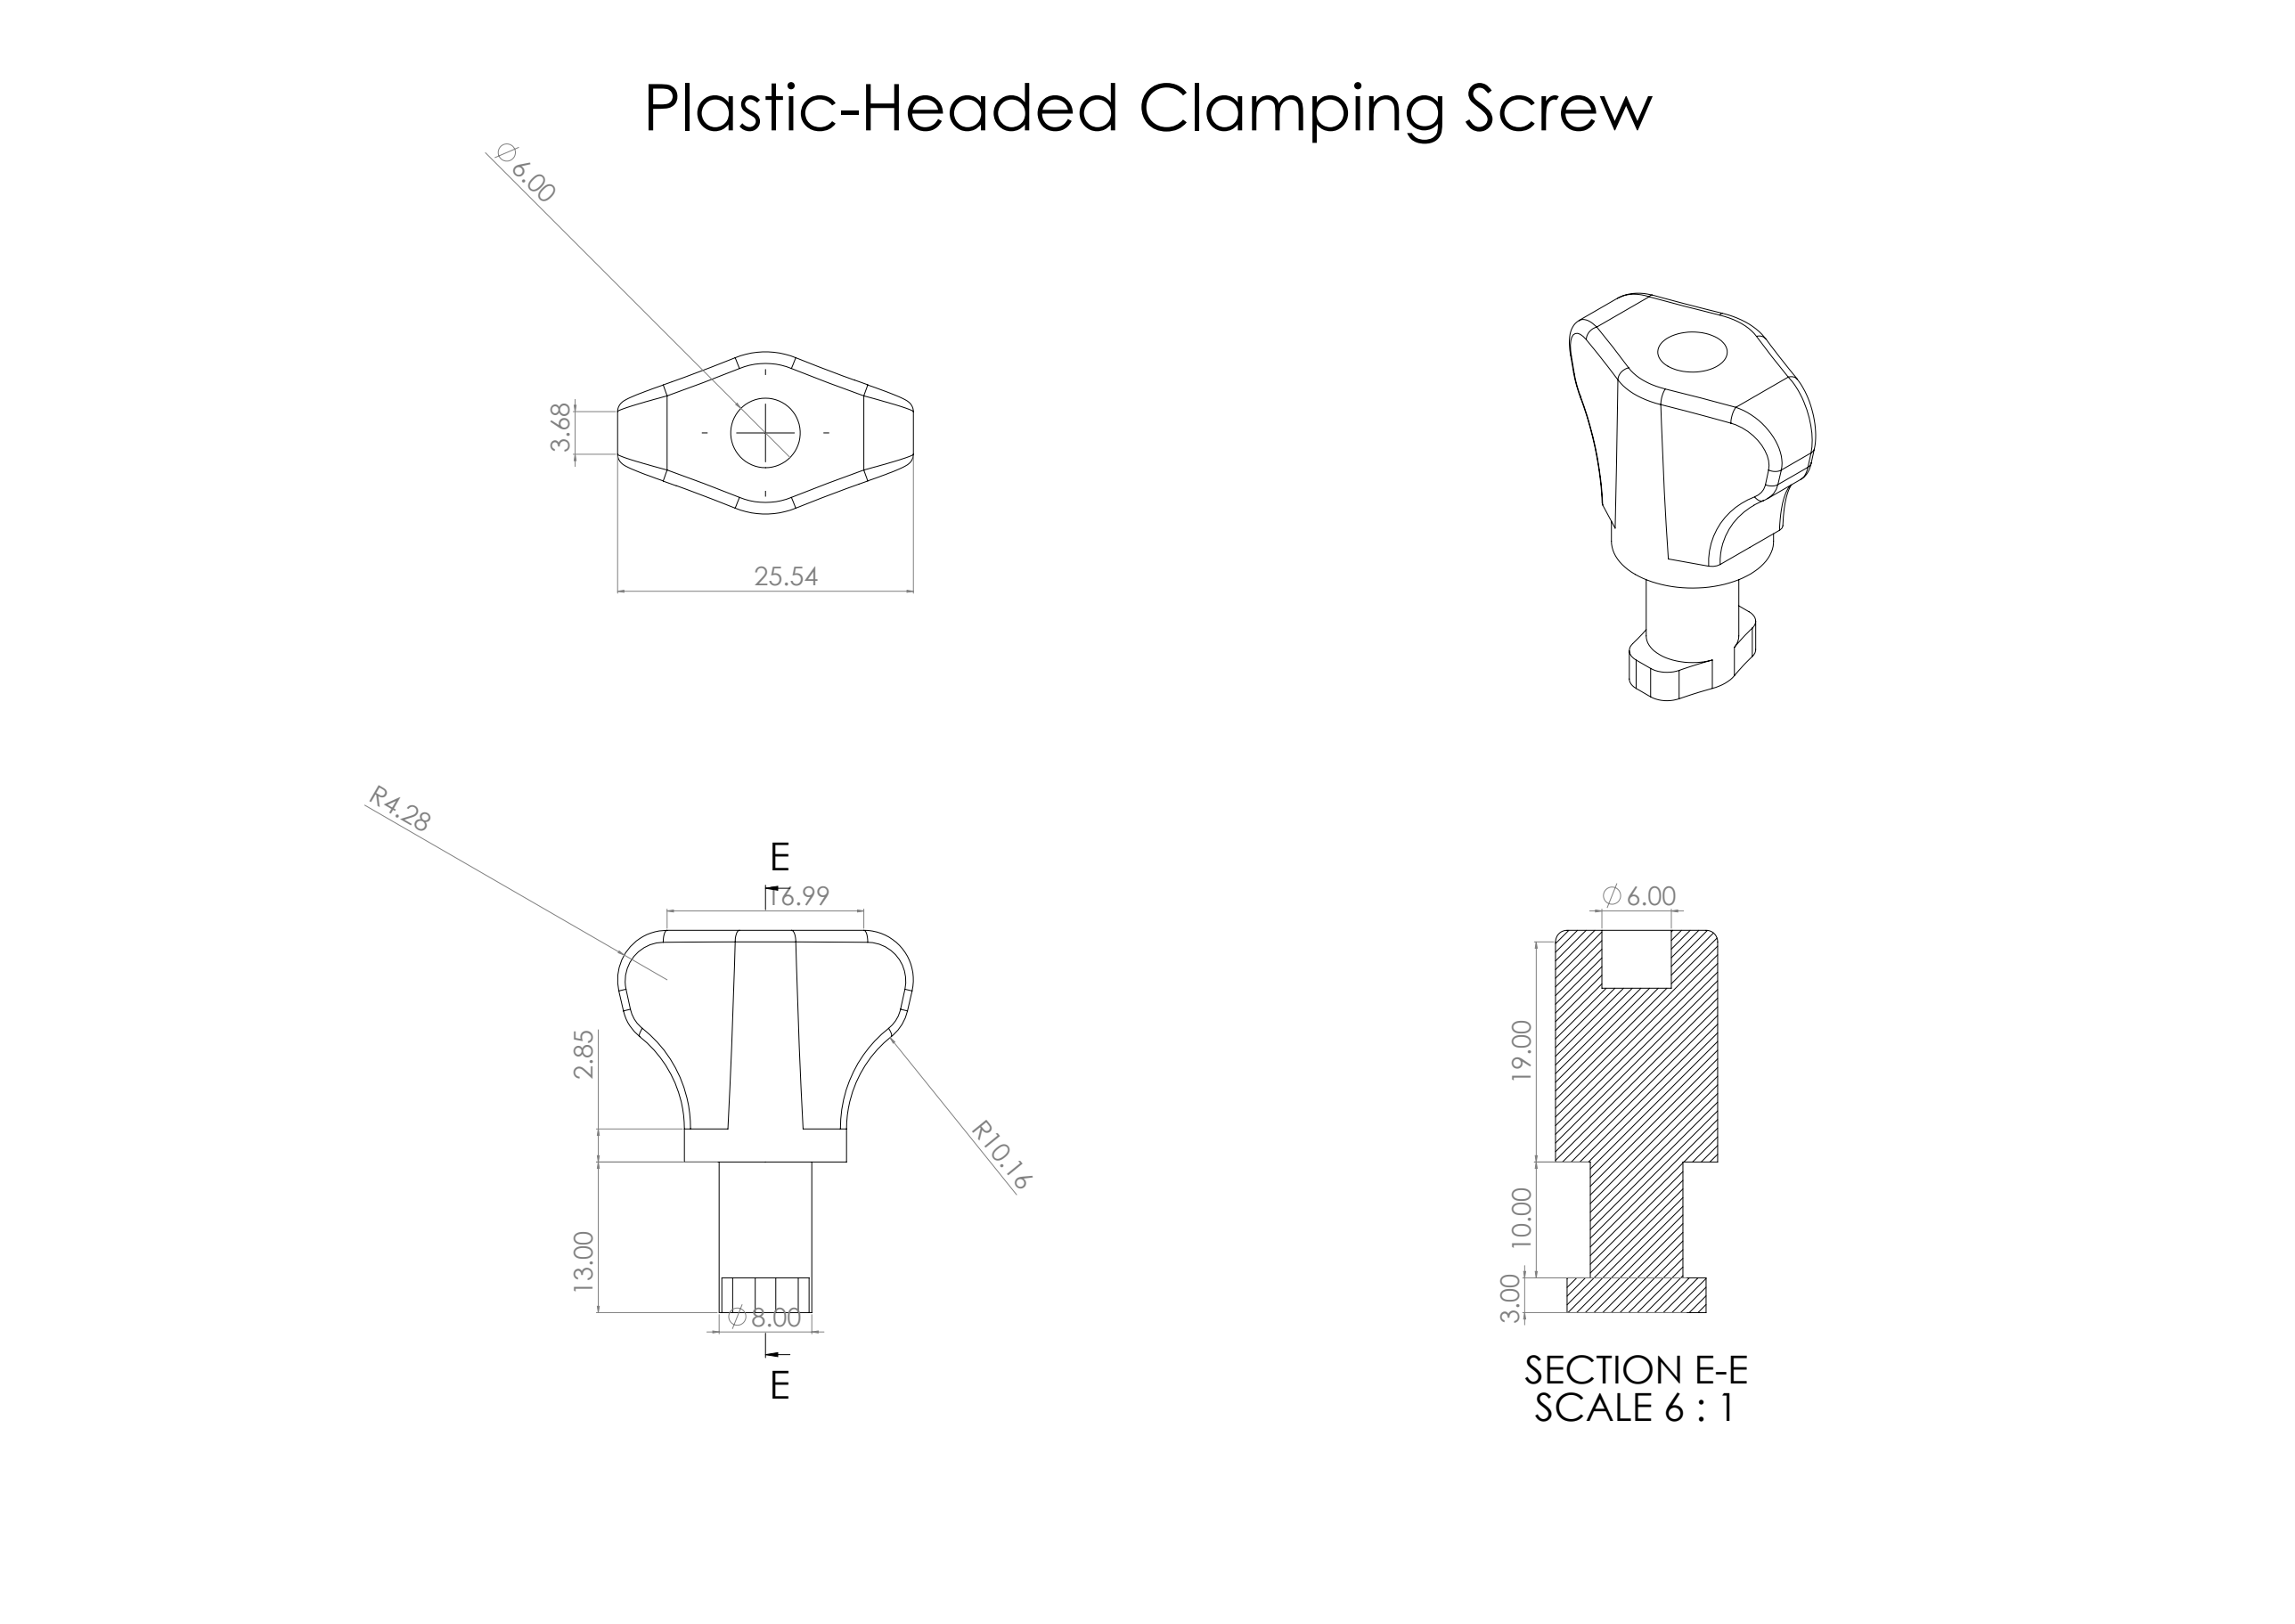
ISO-10303-21;
HEADER;
FILE_DESCRIPTION (('STEP AP214'),
    '1' );
FILE_NAME ('Plastic-Headed Clamping Screw.step',
    '2026-10-24T21:31:31',
    ( '' ),
    ( '' ),
    'SwSTEP 2.0',
    'SolidWorks 2025',
    '' );
FILE_SCHEMA (( 'AUTOMOTIVE_DESIGN' ));
ENDSEC;

DATA;
#4=EDGE_CURVE ( 'NONE', #12159, #10942, #11483, .T. ) ;
#5=EDGE_LOOP ( 'NONE', ( #6099, #8745, #4266, #9000 ) ) ;
#9=CARTESIAN_POINT ( 'NONE',  ( 27.62489819272141389, -52.24929059928630437, 4.899481419381555014 ) ) ;
#10=CARTESIAN_POINT ( 'NONE',  ( 23.72005712271873890, -60.79495753911086098, 6.390225278796987318 ) ) ;
#18=ADVANCED_FACE ( 'NONE', ( #1362 ), #5786, .T. ) ;
#24=ORIENTED_EDGE ( 'NONE', *, *, #9295, .T. ) ;
#52=CARTESIAN_POINT ( 'NONE',  ( 8.091875466796944139, -56.52532528994245808, 1.842181053809107238 ) ) ;
#55=EDGE_CURVE ( 'NONE', #10251, #7651, #14932, .T. ) ;
#67=CARTESIAN_POINT ( 'NONE',  ( 8.466388902489018875, -58.63671300496866223, -1.826958383930360919 ) ) ;
#70=CIRCLE ( 'NONE', #4772, 3.000000000000000888 ) ;
#78=CARTESIAN_POINT ( 'NONE',  ( 10.10272221478045296, -60.61171897230391892, -3.004288329735573804 ) ) ;
#82=B_SPLINE_CURVE_WITH_KNOTS ( 'NONE', 3,
 ( #2803, #3028, #1934, #12180, #8712, #1641, #3094, #13404, #11248, #10961, #410, #7643, #1857, #1791, #7796, #12259, #700, #6406 ),
 .UNSPECIFIED., .F., .F.,
 ( 4, 2, 2, 2, 2, 2, 2, 2, 4 ),
 ( 0.000000000000000000, 0.0007600084067931386217, 0.001520016813586277243, 0.002280025220379415865, 0.003040033627172554487, 0.003800042033965693108, 0.004560050440758831730, 0.005320058847551970352, 0.006080067254345108974 ),
 .UNSPECIFIED. ) ;
#88=FACE_OUTER_BOUND ( 'NONE', #4233, .T. ) ;
#89=ORIENTED_EDGE ( 'NONE', *, *, #5308, .T. ) ;
#91=CARTESIAN_POINT ( 'NONE',  ( 32.77533487224304309, -57.91121052158847249, 2.751677492798574320 ) ) ;
#95=VECTOR ( 'NONE', #9996, 1000.000000000000000 ) ;
#96=DIRECTION ( 'NONE',  ( 0.9421718071228325497, 6.170304995646513309E-16, -0.3351302520855077849 ) ) ;
#102=ORIENTED_EDGE ( 'NONE', *, *, #10358, .T. ) ;
#104=CARTESIAN_POINT ( 'NONE',  ( 9.074528850127588697, -58.48798588983633095, 2.754379989674547780 ) ) ;
#112=EDGE_CURVE ( 'NONE', #12771, #10151, #4658, .T. ) ;
#113=CARTESIAN_POINT ( 'NONE',  ( 33.37135420079148673, -55.04126158147273884, -2.748788379873860599 ) ) ;
#125=CARTESIAN_POINT ( 'NONE',  ( 13.86797143582180780, -68.67521603617343828, 4.260811380360699729 ) ) ;
#126=DIRECTION ( 'NONE',  ( 0.000000000000000000, 0.000000000000000000, 1.000000000000000000 ) ) ;
#129=CARTESIAN_POINT ( 'NONE',  ( 30.58625090343030806, -52.41844408481608752, 2.861639392408844351 ) ) ;
#131=CARTESIAN_POINT ( 'NONE',  ( 20.86173033120691045, -53.24929059928630437, 0.000000000000000000 ) ) ;
#139=CARTESIAN_POINT ( 'NONE',  ( 9.123957934261133218, -53.72645478541605257, 3.103403305059656336 ) ) ;
#143=VERTEX_POINT ( 'NONE', #9046 ) ;
#146=DIRECTION ( 'NONE',  ( -0.9744556954135545901, 0.2245798247307304318, 0.000000000000000000 ) ) ;
#173=CARTESIAN_POINT ( 'NONE',  ( 29.24198010098110245, -64.22824823034754615, 3.135769320951033112 ) ) ;
#174=EDGE_CURVE ( 'NONE', #2378, #7934, #12219, .T. ) ;
#176=CARTESIAN_POINT ( 'NONE',  ( 13.73779544508787431, -66.12426320349668174, 4.110478850042866839 ) ) ;
#180=CARTESIAN_POINT ( 'NONE',  ( 33.55553634841081845, -55.70626543767114214, 1.910065177037574946 ) ) ;
#188=CARTESIAN_POINT ( 'NONE',  ( 18.24487436548682240, -53.24929059928630437, 6.492462156583986399 ) ) ;
#201=CARTESIAN_POINT ( 'NONE',  ( 32.69801279946867112, -53.84541978742783641, 3.062363702218897643 ) ) ;
#226=CYLINDRICAL_SURFACE ( 'NONE', #7156, 10.15857703477299978 ) ;
#228=CARTESIAN_POINT ( 'NONE',  ( 12.36791015745245836, -52.24929059928630437, 3.199931146564424012 ) ) ;
#234=ORIENTED_EDGE ( 'NONE', *, *, #174, .T. ) ;
#239=CARTESIAN_POINT ( 'NONE',  ( 24.10826840236109803, -69.39711819508849544, -6.201611931792124111 ) ) ;
#256=CARTESIAN_POINT ( 'NONE',  ( 9.949736305181877682, -63.13800426656748499, 2.713090553606876121 ) ) ;
#258=CARTESIAN_POINT ( 'NONE',  ( 27.33382790127958728, -69.39711819508849544, 4.502057496415716287 ) ) ;
#259=DIRECTION ( 'NONE',  ( 0.000000000000000000, 0.000000000000000000, 1.000000000000000000 ) ) ;
#261=CARTESIAN_POINT ( 'NONE',  ( 31.94014848486111191, -53.10528739703779877, -3.364210193422788375 ) ) ;
#264=EDGE_CURVE ( 'NONE', #12856, #5130, #362, .T. ) ;
#266=DIRECTION ( 'NONE',  ( -0.000000000000000000, -0.000000000000000000, -1.000000000000000000 ) ) ;
#276=CARTESIAN_POINT ( 'NONE',  ( 31.87918814257875155, -54.14181112192009238, 3.331498666157771016 ) ) ;
#289=CARTESIAN_POINT ( 'NONE',  ( 9.168176149879958103, -53.68423722363644401, 2.283982087543965367 ) ) ;
#300=ORIENTED_EDGE ( 'NONE', *, *, #12912, .T. ) ;
#301=CARTESIAN_POINT ( 'NONE',  ( 13.63336148250377100, -65.27414832489905905, 4.302972696997120039 ) ) ;
#302=VERTEX_POINT ( 'NONE', #4387 ) ;
#304=VERTEX_POINT ( 'NONE', #7858 ) ;
#308=AXIS2_PLACEMENT_3D ( 'NONE', #9751, #6496, #11257 ) ;
#309=ADVANCED_FACE ( 'NONE', ( #12548, #6765 ), #13774, .T. ) ;
#312=CARTESIAN_POINT ( 'NONE',  ( 29.48535251946101710, -62.76259148841303670, -3.786770376139251937 ) ) ;
#314=ORIENTED_EDGE ( 'NONE', *, *, #11289, .T. ) ;
#316=CARTESIAN_POINT ( 'NONE',  ( 32.90197589884652274, -57.33450387999030795, 2.749014434309885235 ) ) ;
#325=ORIENTED_EDGE ( 'NONE', *, *, #6325, .F. ) ;
#330=CARTESIAN_POINT ( 'NONE',  ( 13.85027004230004444, -68.05254135517340330, 4.069129116404105240 ) ) ;
#331=CARTESIAN_POINT ( 'NONE',  ( 32.35433946108159375, -60.80954383512729322, 1.970170733381438222 ) ) ;
#332=VECTOR ( 'NONE', #3067, 1000.000000000000000 ) ;
#333=CARTESIAN_POINT ( 'NONE',  ( 12.03298173962126683, -53.28399145779480506, 4.141535524925028078 ) ) ;
#338=CARTESIAN_POINT ( 'NONE',  ( 32.37230692610057758, -54.69057383521065674, -3.126673503084364203 ) ) ;
#343=DIRECTION ( 'NONE',  ( 0.9744556954135530358, -0.2245798247307378148, 0.000000000000000000 ) ) ;
#362=B_SPLINE_CURVE_WITH_KNOTS ( 'NONE', 3,
 ( #5026, #12249, #5902, #7328, #3856, #12016, #331, #8559, #13257, #9804 ),
 .UNSPECIFIED., .F., .F.,
 ( 4, 2, 2, 2, 4 ),
 ( 0.000000000000000000, 0.0006693228878568694860, 0.001338645775713738972, 0.002007968663570608350, 0.002677291551427477944 ),
 .UNSPECIFIED. ) ;
#374=CARTESIAN_POINT ( 'NONE',  ( 31.12893072306533071, -61.89517205450268733, 2.369674354374375458 ) ) ;
#378=EDGE_LOOP ( 'NONE', ( #12434, #11503, #11290, #1533 ) ) ;
#383=CARTESIAN_POINT ( 'NONE',  ( 19.97461805067967688, 0.000000000000000000, -4.000000000000000888 ) ) ;
#399=CARTESIAN_POINT ( 'NONE',  ( 31.74193665722908264, -52.96285630328479499, 2.532360049841041683 ) ) ;
#407=DIRECTION ( 'NONE',  ( 0.000000000000000000, 0.000000000000000000, 1.000000000000000000 ) ) ;
#410=CARTESIAN_POINT ( 'NONE',  ( 9.212626894557791601, -54.90380519981211194, 3.064473585392920363 ) ) ;
#414=CARTESIAN_POINT ( 'NONE',  ( 27.86173033120691045, -69.39711819508849544, -3.619682905202609380 ) ) ;
#418=ORIENTED_EDGE ( 'NONE', *, *, #1578, .T. ) ;
#420=CARTESIAN_POINT ( 'NONE',  ( 28.47348575918184110, -58.78531205411836424, -4.199849437517832129 ) ) ;
#424=DIRECTION ( 'NONE',  ( 0.000000000000000000, 0.000000000000000000, -1.000000000000000000 ) ) ;
#425=DIRECTION ( 'NONE',  ( 0.000000000000000000, -1.000000000000000000, 0.000000000000000000 ) ) ;
#427=ORIENTED_EDGE ( 'NONE', *, *, #10079, .F. ) ;
#430=ADVANCED_FACE ( 'NONE', ( #12701 ), #5856, .T. ) ;
#432=CYLINDRICAL_SURFACE ( 'NONE', #9177, 3.951771890309582869 ) ;
#439=LINE ( 'NONE', #4985, #3268 ) ;
#447=CARTESIAN_POINT ( 'NONE',  ( 28.71810018070638648, -65.29678988936899486, 3.348867343503173721 ) ) ;
#448=ADVANCED_FACE ( 'NONE', ( #7159 ), #15184, .T. ) ;
#462=ORIENTED_EDGE ( 'NONE', *, *, #9510, .T. ) ;
#463=EDGE_LOOP ( 'NONE', ( #8239, #3179, #633, #6797, #6640 ) ) ;
#468=( BOUNDED_SURFACE ( )  B_SPLINE_SURFACE ( 3, 2, ( 
 ( #9739, #10958, #7416 ),
 ( #11029, #14423, #4081 ),
 ( #12112, #6268, #3867 ),
 ( #14564, #12255, #11095 ) ),
 .UNSPECIFIED., .F., .F., .F. ) 
 B_SPLINE_SURFACE_WITH_KNOTS ( ( 4, 4 ),
 ( 3, 3 ),
 ( 0.000000000000000000, 0.001771943201165730557 ),
 ( 0.000000000000000000, 1.000000000000000000 ),
 .UNSPECIFIED. ) 
 GEOMETRIC_REPRESENTATION_ITEM ( )  RATIONAL_B_SPLINE_SURFACE ( (
 ( 1.000000000000000000, 0.8308543624379411963, 1.000000000000000000),
 ( 1.000000000000000000, 0.8288551047899443969, 1.000000000000000000),
 ( 1.000000000000000000, 0.8269348987755755775, 1.000000000000000000),
 ( 1.000000000000000000, 0.8250833044923659987, 1.000000000000000000) ) ) 
 REPRESENTATION_ITEM ( '' )  SURFACE ( )  );
#470=CARTESIAN_POINT ( 'NONE',  ( 10.05209847106513621, -63.64501252278640919, 2.710939438195351325 ) ) ;
#474=CARTESIAN_POINT ( 'NONE',  ( 13.86142555056148851, -69.48056866272027321, -4.214447830835809761 ) ) ;
#484=DIRECTION ( 'NONE',  ( 0.3351302520855081735, 0.000000000000000000, -0.9421718071228324387 ) ) ;
#500=CARTESIAN_POINT ( 'NONE',  ( 29.27360327072251067, -58.32476007869853873, 2.500000000000000000 ) ) ;
#502=CARTESIAN_POINT ( 'NONE',  ( 20.86173033120691045, -72.24929059928631148, 3.999999999999999112 ) ) ;
#508=AXIS2_PLACEMENT_3D ( 'NONE', #2758, #1819, #6294 ) ;
#512=CARTESIAN_POINT ( 'NONE',  ( 27.33509234239454244, -69.49659648540917090, 4.497058153269692937 ) ) ;
#544=CARTESIAN_POINT ( 'NONE',  ( 10.45251858056743011, -61.76394201830515129, -3.065891788180099553 ) ) ;
#552=DIRECTION ( 'NONE',  ( -0.2245798247307348172, -0.9744556954135535909, 0.000000000000000000 ) ) ;
#554=( NAMED_UNIT ( * ) PLANE_ANGLE_UNIT ( ) SI_UNIT ( $, .RADIAN. ) );
#564=CARTESIAN_POINT ( 'NONE',  ( 20.86173033120691045, -57.24929059928630437, 0.000000000000000000 ) ) ;
#567=CARTESIAN_POINT ( 'NONE',  ( 23.50212160826626118, -54.09900330347249309, -6.482993899729486920 ) ) ;
#572=DIRECTION ( 'NONE',  ( 0.000000000000000000, 0.000000000000000000, -1.000000000000000000 ) ) ;
#574=ORIENTED_EDGE ( 'NONE', *, *, #3154, .F. ) ;
#579=CARTESIAN_POINT ( 'NONE',  ( 11.75462132594869047, -63.18892729117109042, 3.546101824479054976 ) ) ;
#580=EDGE_CURVE ( 'NONE', #13749, #4765, #2911, .T. ) ;
#581=CARTESIAN_POINT ( 'NONE',  ( 11.41483174849314786, -52.33251913750716255, 3.960984348906031460 ) ) ;
#585=FACE_OUTER_BOUND ( 'NONE', #3678, .T. ) ;
#598=FACE_OUTER_BOUND ( 'NONE', #463, .T. ) ;
#599=CYLINDRICAL_SURFACE ( 'NONE', #8676, 10.15857703477299623 ) ;
#611=CARTESIAN_POINT ( 'NONE',  ( 8.749277640414614865, -56.32592369292856915, -2.799485268159552120 ) ) ;
#615=CARTESIAN_POINT ( 'NONE',  ( 14.40311142432127056, -68.64054039872911517, -4.542265185092021262 ) ) ;
#617=CARTESIAN_POINT ( 'NONE',  ( 33.62912904389242641, -56.86646964060239640, 2.513983171436027231 ) ) ;
#621=FACE_OUTER_BOUND ( 'NONE', #8917, .T. ) ;
#622=EDGE_CURVE ( 'NONE', #15091, #1508, #10780, .T. ) ;
#624=CARTESIAN_POINT ( 'NONE',  ( 9.200644618036296407, -59.06479067038043240, -2.757123406423053424 ) ) ;
#625=VERTEX_POINT ( 'NONE', #1612 ) ;
#627=CARTESIAN_POINT ( 'NONE',  ( 27.86173033120691045, -69.39711819508848123, -3.801276035476822468 ) ) ;
#632=CARTESIAN_POINT ( 'NONE',  ( 28.15780090692999593, -63.36830850591302067, -4.156137255743351133 ) ) ;
#633=ORIENTED_EDGE ( 'NONE', *, *, #14074, .F. ) ;
#640=CIRCLE ( 'NONE', #11212, 0.9999999999999996669 ) ;
#643=CARTESIAN_POINT ( 'NONE',  ( 31.33007899711186894, -52.72918400488543256, -2.651310087704546348 ) ) ;
#651=AXIS2_PLACEMENT_3D ( 'NONE', #8278, #11802, #11951 ) ;
#652=DIRECTION ( 'NONE',  ( 0.000000000000000000, 0.000000000000000000, -1.000000000000000000 ) ) ;
#656=EDGE_LOOP ( 'NONE', ( #5765, #14402, #234, #3280, #10430, #12233, #7508, #462, #7848 ) ) ;
#658=B_SPLINE_CURVE_WITH_KNOTS ( 'NONE', 3,
 ( #10135, #10365, #13747, #3202 ),
 .UNSPECIFIED., .F., .F.,
 ( 4, 4 ),
 ( 0.000000000000000000, 0.001771361151111829372 ),
 .UNSPECIFIED. ) ;
#662=ORIENTED_EDGE ( 'NONE', *, *, #7032, .T. ) ;
#666=ORIENTED_EDGE ( 'NONE', *, *, #12524, .F. ) ;
#668=CARTESIAN_POINT ( 'NONE',  ( 11.71690433395004227, -52.27452423507673274, -4.068013018868786190 ) ) ;
#669=DIRECTION ( 'NONE',  ( -0.6198786537240911221, -0.7846976836063734861, 0.000000000000000000 ) ) ;
#672=ORIENTED_EDGE ( 'NONE', *, *, #12291, .F. ) ;
#680=CARTESIAN_POINT ( 'NONE',  ( 8.597635011448854669, -59.20619211347771227, -2.502190571104482952 ) ) ;
#684=EDGE_CURVE ( 'NONE', #12779, #2517, #9724, .T. ) ;
#688=CARTESIAN_POINT ( 'NONE',  ( 12.06814882729969440, -63.62021712492819603, -2.966460067268481549 ) ) ;
#694=ORIENTED_EDGE ( 'NONE', *, *, #1475, .T. ) ;
#700=CARTESIAN_POINT ( 'NONE',  ( 8.766252841628377368, -57.08298494442340143, 2.747852995220871009 ) ) ;
#701=CARTESIAN_POINT ( 'NONE',  ( 10.00023835250150483, -61.42570632716525125, 2.132522520905371977 ) ) ;
#704=AXIS2_PLACEMENT_3D ( 'NONE', #10886, #8709, #343 ) ;
#710=ORIENTED_EDGE ( 'NONE', *, *, #1180, .T. ) ;
#716=CARTESIAN_POINT ( 'NONE',  ( 14.22956937301584546, -69.39711819508849544, -4.416273062436609109 ) ) ;
#720=CARTESIAN_POINT ( 'NONE',  ( 8.649830367478799076, -59.43266865480772054, -1.834006918418332521 ) ) ;
#728=DIRECTION ( 'NONE',  ( 0.000000000000000000, 1.000000000000000000, 0.000000000000000000 ) ) ;
#736=ORIENTED_EDGE ( 'NONE', *, *, #1578, .F. ) ;
#743=DIRECTION ( 'NONE',  ( -0.000000000000000000, -0.000000000000000000, -1.000000000000000000 ) ) ;
#753=EDGE_CURVE ( 'NONE', #12307, #1292, #9416, .T. ) ;
#759=LINE ( 'NONE', #8997, #13503 ) ;
#764=CARTESIAN_POINT ( 'NONE',  ( 15.46081644285382772, -69.39711819508849544, 5.076148092048922145 ) ) ;
#768=CARTESIAN_POINT ( 'NONE',  ( 32.90197589884652274, -57.33450387999031506, 2.749014434309864363 ) ) ;
#773=CARTESIAN_POINT ( 'NONE',  ( 29.49975272800921289, -62.74348037527474276, -3.781439773221457301 ) ) ;
#783=CARTESIAN_POINT ( 'NONE',  ( 32.95707784766408110, -57.08357682498795072, 2.747855728348003179 ) ) ;
#790=CIRCLE ( 'NONE', #3744, 2.000000000000000000 ) ;
#792=CARTESIAN_POINT ( 'NONE',  ( 20.86173033120691045, -57.24929059928630437, 3.000000000000000888 ) ) ;
#797=CIRCLE ( 'NONE', #14087, 1.000000000000001332 ) ;
#798=CARTESIAN_POINT ( 'NONE',  ( 13.51972775594646947, -66.75404937493283342, 3.551013195535614120 ) ) ;
#801=CARTESIAN_POINT ( 'NONE',  ( 33.59633122631266389, -57.16466038563396523, -1.814534822646767909 ) ) ;
#808=CARTESIAN_POINT ( 'NONE',  ( 7.497055383622185154, -51.17811635675307969, -2.733205671937324777 ) ) ;
#811=ORIENTED_EDGE ( 'NONE', *, *, #7029, .T. ) ;
#814=ADVANCED_FACE ( 'NONE', ( #10570 ), #5184, .T. ) ;
#816=DIRECTION ( 'NONE',  ( 0.000000000000000000, 0.000000000000000000, -1.000000000000000000 ) ) ;
#822=CARTESIAN_POINT ( 'NONE',  ( 8.605785544313173219, -54.47948885957401188, -2.876625435111462625 ) ) ;
#829=EDGE_LOOP ( 'NONE', ( #10229, #6980, #7558, #1341 ) ) ;
#832=EDGE_LOOP ( 'NONE', ( #908, #9068, #8291, #12526 ) ) ;
#834=FACE_OUTER_BOUND ( 'NONE', #12615, .T. ) ;
#835=CARTESIAN_POINT ( 'NONE',  ( 10.21509949969620834, -53.84182990103197142, -3.477143273224481579 ) ) ;
#840=CARTESIAN_POINT ( 'NONE',  ( 32.90197589884652274, -57.33450387999030085, -2.749014434309871024 ) ) ;
#843=ADVANCED_FACE ( 'NONE', ( #8557 ), #10988, .F. ) ;
#849=CARTESIAN_POINT ( 'NONE',  ( 27.69711443911335991, -66.46764508687284945, -4.441229594909795964 ) ) ;
#853=B_SPLINE_CURVE_WITH_KNOTS ( 'NONE', 3,
 ( #870, #3338, #5576, #8037, #7337, #2342 ),
 .UNSPECIFIED., .F., .F.,
 ( 4, 2, 4 ),
 ( 0.000000000000000000, 0.008081365602589977992, 0.01616273120517995598 ),
 .UNSPECIFIED. ) ;
#867=CARTESIAN_POINT ( 'NONE',  ( 27.90872427450967663, -67.42803803071015523, -4.083598241683256802 ) ) ;
#870=CARTESIAN_POINT ( 'NONE',  ( 24.10826840236108737, -69.39711819508849544, 6.201611931792130328 ) ) ;
#876=CARTESIAN_POINT ( 'NONE',  ( 30.90164406145839138, -52.52607756353321378, -2.773424542755355660 ) ) ;
#880=CARTESIAN_POINT ( 'NONE',  ( 17.58146340911262584, -70.03159917003323187, -6.184016381205385215 ) ) ;
#881=EDGE_CURVE ( 'NONE', #5130, #10222, #5376, .T. ) ;
#882=EDGE_CURVE ( 'NONE', #9663, #7432, #3526, .T. ) ;
#883=ORIENTED_EDGE ( 'NONE', *, *, #13767, .T. ) ;
#884=CARTESIAN_POINT ( 'NONE',  ( 8.201103799357262858, -57.48563641131178770, 1.816685854991387794 ) ) ;
#897=CARTESIAN_POINT ( 'NONE',  ( 8.615075654522891924, -54.46933172536110845, -2.097670533079140309 ) ) ;
#908=ORIENTED_EDGE ( 'NONE', *, *, #2368, .F. ) ;
#911=CARTESIAN_POINT ( 'NONE',  ( 9.654882263607307280, -61.15288932781407283, -2.038807541293268688 ) ) ;
#913=CARTESIAN_POINT ( 'NONE',  ( 11.08356997321305393, -53.42334933900650640, -3.800563870772192043 ) ) ;
#918=CARTESIAN_POINT ( 'NONE',  ( 33.63443549450521175, -56.24768769701492488, -2.562823873651032258 ) ) ;
#919=CARTESIAN_POINT ( 'NONE',  ( 27.60269520869854887, -53.27034158699149913, 4.884662653952318578 ) ) ;
#920=CARTESIAN_POINT ( 'NONE',  ( 32.22669677403312960, -60.90158242457943771, 2.720958399978099074 ) ) ;
#921=VECTOR ( 'NONE', #8754, 1000.000000000000000 ) ;
#926=ADVANCED_FACE ( 'NONE', ( #10219 ), #599, .F. ) ;
#939=ORIENTED_EDGE ( 'NONE', *, *, #13244, .T. ) ;
#942=VECTOR ( 'NONE', #14321, 1000.000000000000000 ) ;
#945=CARTESIAN_POINT ( 'NONE',  ( 11.00552470667372340, -52.46278122153624679, 2.824859710458689666 ) ) ;
#946=ORIENTED_EDGE ( 'NONE', *, *, #10645, .T. ) ;
#955=CARTESIAN_POINT ( 'NONE',  ( 31.49298359385885959, -60.71197230342421136, 3.050751728647414840 ) ) ;
#967=LINE ( 'NONE', #2211, #12353 ) ;
#972=CARTESIAN_POINT ( 'NONE',  ( 10.86432672294017365, -53.50034303113530143, -3.720434809418780908 ) ) ;
#987=EDGE_CURVE ( 'NONE', #7237, #11741, #11214, .T. ) ;
#997=CARTESIAN_POINT ( 'NONE',  ( 17.09549820959326638, -85.24929059928631148, 1.347403282660979640 ) ) ;
#998=CARTESIAN_POINT ( 'NONE',  ( 18.24487436548682240, -53.24929059928630437, 6.492462156583975741 ) ) ;
#1015=CARTESIAN_POINT ( 'NONE',  ( 31.88839645113984034, -54.14139889408636463, 3.328424545751987651 ) ) ;
#1025=CARTESIAN_POINT ( 'NONE',  ( 8.233817939642571915, -55.39655954610098121, 1.945404611338338974 ) ) ;
#1032=CIRCLE ( 'NONE', #3494, 1.000000000000000000 ) ;
#1034=CARTESIAN_POINT ( 'NONE',  ( 20.86173033120691045, -52.24929059928630437, 0.000000000000000000 ) ) ;
#1036=CARTESIAN_POINT ( 'NONE',  ( 20.86173033120691045, -72.24929059928631148, -7.000000000000000000 ) ) ;
#1044=CARTESIAN_POINT ( 'NONE',  ( 9.843069943267799715, -62.60658208063265562, -2.715520055324554427 ) ) ;
#1059=CARTESIAN_POINT ( 'NONE',  ( 10.02953924049373313, -52.92218391219020646, -3.457912412237230892 ) ) ;
#1062=ORIENTED_EDGE ( 'NONE', *, *, #6313, .F. ) ;
#1063=CARTESIAN_POINT ( 'NONE',  ( 33.25707175992483400, -58.63671300496854144, 1.826958383950116671 ) ) ;
#1089=VERTEX_POINT ( 'NONE', #3597 ) ;
#1092=CARTESIAN_POINT ( 'NONE',  ( 8.700857908379099115, -59.65407802634350531, 1.835581805806634215 ) ) ;
#1102=CARTESIAN_POINT ( 'NONE',  ( 32.05792886619255455, -60.12744825561602369, -2.859530283892876668 ) ) ;
#1105=CARTESIAN_POINT ( 'NONE',  ( 23.47858629692699139, -53.24929059928630437, 6.492462156583989064 ) ) ;
#1107=CARTESIAN_POINT ( 'NONE',  ( 24.62796245282055452, -96.56299909827106376, -1.347403282660978752 ) ) ;
#1109=CARTESIAN_POINT ( 'NONE',  ( 24.62796245282055452, -85.24929059928631148, 1.347403282660977641 ) ) ;
#1111=VERTEX_POINT ( 'NONE', #2446 ) ;
#1112=CARTESIAN_POINT ( 'NONE',  ( 12.65255919500326165, -50.97757525706221315, -4.214488946479060694 ) ) ;
#1113=EDGE_LOOP ( 'NONE', ( #12679, #6087, #3200, #7335 ) ) ;
#1116=CARTESIAN_POINT ( 'NONE',  ( 14.03037318137822886, -66.48338622332325087, -4.442552071294021410 ) ) ;
#1130=EDGE_CURVE ( 'NONE', #10151, #9216, #11372, .T. ) ;
#1131=EDGE_CURVE ( 'NONE', #7651, #2922, #2136, .T. ) ;
#1134=FACE_OUTER_BOUND ( 'NONE', #14394, .T. ) ;
#1145=ADVANCED_FACE ( 'NONE', ( #4680 ), #2298, .T. ) ;
#1155=CARTESIAN_POINT ( 'NONE',  ( 27.90816809802827692, -67.42878071151913844, 4.083908651743608509 ) ) ;
#1160=VECTOR ( 'NONE', #10730, 1000.000000000000000 ) ;
#1163=CARTESIAN_POINT ( 'NONE',  ( 18.61871093201826355, -53.24929059928630437, 5.564967562786272914 ) ) ;
#1166=PLANE ( 'NONE',  #9038 ) ;
#1180=EDGE_CURVE ( 'NONE', #11520, #11986, #1561, .T. ) ;
#1188=CARTESIAN_POINT ( 'NONE',  ( 18.16985775135671943, -55.94205978621073427, 6.462225911923643373 ) ) ;
#1193=CARTESIAN_POINT ( 'NONE',  ( 13.86584091103555139, -68.67486713609712012, 3.656664647209427521 ) ) ;
#1194=EDGE_CURVE ( 'NONE', #9216, #11968, #7461, .T. ) ;
#1200=CARTESIAN_POINT ( 'NONE',  ( 13.86173033120691223, -69.39711819508849544, 3.619682905202618262 ) ) ;
#1201=CARTESIAN_POINT ( 'NONE',  ( 32.13751574144283296, -54.40403913628106380, 3.226152465599038344 ) ) ;
#1203=ORIENTED_EDGE ( 'NONE', *, *, #14249, .T. ) ;
#1208=CARTESIAN_POINT ( 'NONE',  ( 21.74884261173415467, -96.56299909827106376, -4.000000000000000888 ) ) ;
#1221=ORIENTED_EDGE ( 'NONE', *, *, #8483, .F. ) ;
#1236=EDGE_CURVE ( 'NONE', #11968, #14491, #439, .T. ) ;
#1247=CARTESIAN_POINT ( 'NONE',  ( 32.87486430914729141, -60.00492685494704403, -2.531405393170241158 ) ) ;
#1249=CARTESIAN_POINT ( 'NONE',  ( 28.08719811482655970, -65.28118056119629387, 4.304032224033948140 ) ) ;
#1250=CARTESIAN_POINT ( 'NONE',  ( 14.46725369622999402, -52.24929059928630437, -3.946667064627067845 ) ) ;
#1251=CARTESIAN_POINT ( 'NONE',  ( 31.16509434949074731, -52.62744651407953000, -3.653242136006408014 ) ) ;
#1258=CARTESIAN_POINT ( 'NONE',  ( 17.87818865416385705, -64.01730164816845559, 6.333338579777398891 ) ) ;
#1265=EDGE_LOOP ( 'NONE', ( #4395, #8035, #13913, #9464 ) ) ;
#1270=CARTESIAN_POINT ( 'NONE',  ( 33.43717902155964339, -55.20947656326173103, 1.969991847668780993 ) ) ;
#1278=DIRECTION ( 'NONE',  ( -0.000000000000000000, 1.000000000000000000, -0.000000000000000000 ) ) ;
#1283=CARTESIAN_POINT ( 'NONE',  ( 9.670226323787769473, -54.31204422905957330, 3.261005077968429422 ) ) ;
#1286=DIRECTION ( 'NONE',  ( 0.000000000000000000, -1.000000000000000000, 0.000000000000000000 ) ) ;
#1292=VERTEX_POINT ( 'NONE', #502 ) ;
#1305=DIRECTION ( 'NONE',  ( 0.000000000000000000, 0.000000000000000000, -1.000000000000000000 ) ) ;
#1318=ORIENTED_EDGE ( 'NONE', *, *, #5485, .T. ) ;
#1331=CARTESIAN_POINT ( 'NONE',  ( 31.49298359385885959, -60.71197230342421136, 3.050751728647414840 ) ) ;
#1333=CARTESIAN_POINT ( 'NONE',  ( 32.86037637810374434, -54.05488119003602776, -2.185023599737637490 ) ) ;
#1341=ORIENTED_EDGE ( 'NONE', *, *, #987, .F. ) ;
#1349=EDGE_CURVE ( 'NONE', #4027, #4392, #4504, .T. ) ;
#1351=ORIENTED_EDGE ( 'NONE', *, *, #12911, .T. ) ;
#1362=FACE_OUTER_BOUND ( 'NONE', #1607, .T. ) ;
#1363=DIRECTION ( 'NONE',  ( 0.000000000000000000, 0.000000000000000000, 1.000000000000000000 ) ) ;
#1365=EDGE_CURVE ( 'NONE', #8543, #4896, #11578, .T. ) ;
#1371=CARTESIAN_POINT ( 'NONE',  ( 12.91143137450191247, -63.78335865426897300, 4.036657210498128201 ) ) ;
#1373=CARTESIAN_POINT ( 'NONE',  ( 14.12076545371521519, -53.27034158699100175, 4.884662653952321243 ) ) ;
#1392=FACE_OUTER_BOUND ( 'NONE', #11151, .T. ) ;
#1400=CARTESIAN_POINT ( 'NONE',  ( 9.495483015351213751, -60.90019506145881678, 2.720530867599800562 ) ) ;
#1405=CARTESIAN_POINT ( 'NONE',  ( 33.46718823248610875, -55.33425260370049870, -2.693485533442558033 ) ) ;
#1410=EDGE_LOOP ( 'NONE', ( #8484, #1826, #6584, #10863 ) ) ;
#1411=DIRECTION ( 'NONE',  ( 0.000000000000000000, 0.000000000000000000, -1.000000000000000000 ) ) ;
#1412=CARTESIAN_POINT ( 'NONE',  ( 32.31153295206774345, -59.69665779701220032, -2.790274538705360019 ) ) ;
#1424=CARTESIAN_POINT ( 'NONE',  ( 32.75756170203653284, -53.92993659400953277, 2.218374547572117716 ) ) ;
#1434=CARTESIAN_POINT ( 'NONE',  ( 32.90197589884652274, -57.33450387999030795, -2.749014434309867916 ) ) ;
#1440=ORIENTED_EDGE ( 'NONE', *, *, #2063, .F. ) ;
#1442=CARTESIAN_POINT ( 'NONE',  ( 8.406258358832010558, -54.90785108970787576, 2.018552575025332363 ) ) ;
#1451=CARTESIAN_POINT ( 'NONE',  ( 27.60446587309679956, -53.27035316348869998, 4.884032402486375268 ) ) ;
#1463=AXIS2_PLACEMENT_3D ( 'NONE', #12026, #14631, #552 ) ;
#1475=EDGE_CURVE ( 'NONE', #2336, #8264, #13597, .T. ) ;
#1477=CARTESIAN_POINT ( 'NONE',  ( 8.199792978590130232, -57.47994873761393109, 2.501453769636607039 ) ) ;
#1481=CARTESIAN_POINT ( 'NONE',  ( 18.13205847682796090, -57.03285117767145351, 6.445925775545124914 ) ) ;
#1486=CARTESIAN_POINT ( 'NONE',  ( 31.69252035015315627, -52.93050895625588481, -3.457921359511734849 ) ) ;
#1487=B_SPLINE_CURVE_WITH_KNOTS ( 'NONE', 3,
 ( #955, #15051, #12505, #10283, #5585, #3191, #11341, #12663, #7819, #14971 ),
 .UNSPECIFIED., .F., .F.,
 ( 4, 2, 2, 2, 4 ),
 ( 0.000000000000000000, 0.0004999547661763323846, 0.0009999095323526647691, 0.001499864298528997154, 0.001999819064705329538 ),
 .UNSPECIFIED. ) ;
#1495=CIRCLE ( 'NONE', #10091, 2.000000000000000000 ) ;
#1503=ORIENTED_EDGE ( 'NONE', *, *, #6773, .T. ) ;
#1508=VERTEX_POINT ( 'NONE', #5589 ) ;
#1512=DIRECTION ( 'NONE',  ( 0.000000000000000000, -1.000000000000000000, 0.000000000000000000 ) ) ;
#1513=AXIS2_PLACEMENT_3D ( 'NONE', #564, #3097, #1718 ) ;
#1514=CIRCLE ( 'NONE', #8871, 2.000000000000000000 ) ;
#1517=CARTESIAN_POINT ( 'NONE',  ( 8.129887667336562984, -57.17459804181999772, 2.501046471591553466 ) ) ;
#1518=EDGE_CURVE ( 'NONE', #5832, #10536, #14827, .T. ) ;
#1532=CARTESIAN_POINT ( 'NONE',  ( 30.59344312246462394, -62.42480215138191113, 2.585081138710340731 ) ) ;
#1533=ORIENTED_EDGE ( 'NONE', *, *, #8483, .T. ) ;
#1540=CARTESIAN_POINT ( 'NONE',  ( 28.60124718008471234, -65.57050171853261133, -4.044987206835048532 ) ) ;
#1542=CARTESIAN_POINT ( 'NONE',  ( 26.26264421955999140, -69.39711819508849544, -5.076148092048929250 ) ) ;
#1558=DIRECTION ( 'NONE',  ( 0.000000000000000000, -1.000000000000000000, 0.000000000000000000 ) ) ;
#1560=CARTESIAN_POINT ( 'NONE',  ( 12.72502611717542109, -51.89470720432451145, 4.215327498671517681 ) ) ;
#1561=CIRCLE ( 'NONE', #6462, 7.000000000000000000 ) ;
#1565=CARTESIAN_POINT ( 'NONE',  ( 32.09878978612020006, -53.24145049768157634, -2.425475548245525470 ) ) ;
#1569=ORIENTED_EDGE ( 'NONE', *, *, #12912, .F. ) ;
#1572=CARTESIAN_POINT ( 'NONE',  ( 17.61519226005271577, -69.39711819508849544, 6.201611931792121446 ) ) ;
#1578=EDGE_CURVE ( 'NONE', #10002, #10908, #7906, .T. ) ;
#1591=CARTESIAN_POINT ( 'NONE',  ( 9.216223969337589139, -54.89772082965570377, 3.066133849897938468 ) ) ;
#1592=DIRECTION ( 'NONE',  ( 1.734723475976807094E-15, 0.000000000000000000, -1.000000000000000000 ) ) ;
#1596=CARTESIAN_POINT ( 'NONE',  ( 8.599030766203958009, -59.21224831720011395, 2.500000000000000000 ) ) ;
#1597=ADVANCED_FACE ( 'NONE', ( #2113 ), #10588, .F. ) ;
#1607=EDGE_LOOP ( 'NONE', ( #662, #7615, #7842, #2669, #7464 ) ) ;
#1608=CARTESIAN_POINT ( 'NONE',  ( 28.20373290646802289, -66.75404937492989177, -3.551013195539084677 ) ) ;
#1612=CARTESIAN_POINT ( 'NONE',  ( 21.74884261173415467, -85.24929059928631148, -6.000000000000000888 ) ) ;
#1616=CYLINDRICAL_SURFACE ( 'NONE', #11018, 31.00000000000000000 ) ;
#1627=CARTESIAN_POINT ( 'NONE',  ( 17.45100281819997079, -72.28366650274460881, 6.113054590623445250 ) ) ;
#1631=CARTESIAN_POINT ( 'NONE',  ( 14.38836832001927846, -69.49659648540917090, -4.497058153269694714 ) ) ;
#1641=CARTESIAN_POINT ( 'NONE',  ( 10.42210623299234840, -53.71252461569496006, 3.555803702006939737 ) ) ;
#1646=CARTESIAN_POINT ( 'NONE',  ( 27.48632486622552662, -69.39711819508849544, -4.406545790198922674 ) ) ;
#1647=CARTESIAN_POINT ( 'NONE',  ( 8.333746554286264541, -58.06117559053629407, -1.821720188324787992 ) ) ;
#1652=AXIS2_PLACEMENT_3D ( 'NONE', #7089, #5870, #4698 ) ;
#1653=ORIENTED_EDGE ( 'NONE', *, *, #4198, .F. ) ;
#1655=DIRECTION ( 'NONE',  ( -0.000000000000000000, 1.000000000000000000, -0.000000000000000000 ) ) ;
#1665=DIRECTION ( 'NONE',  ( 0.000000000000000000, -1.000000000000000000, 0.000000000000000000 ) ) ;
#1666=AXIS2_PLACEMENT_3D ( 'NONE', #14514, #1665, #8887 ) ;
#1678=CARTESIAN_POINT ( 'NONE',  ( 17.09549820959326638, -82.24929059928629727, -1.347403282660980528 ) ) ;
#1681=CARTESIAN_POINT ( 'NONE',  ( 23.36173033120691400, -82.24929059928629727, 6.000000000000001776 ) ) ;
#1694=EDGE_CURVE ( 'NONE', #1089, #7432, #9259, .T. ) ;
#1703=CARTESIAN_POINT ( 'NONE',  ( 14.38963276113423895, -69.39711819508849544, 4.502057496415707405 ) ) ;
#1704=CARTESIAN_POINT ( 'NONE',  ( 18.03113812440136243, 0.000000000000000000, -4.472107801411127959 ) ) ;
#1710=FACE_OUTER_BOUND ( 'NONE', #11202, .T. ) ;
#1713=CARTESIAN_POINT ( 'NONE',  ( 33.25707175001029015, -58.63671304798791084, -1.826958385055442058 ) ) ;
#1715=CIRCLE ( 'NONE', #13510, 6.000000000000000000 ) ;
#1718=DIRECTION ( 'NONE',  ( 0.000000000000000000, 0.000000000000000000, 1.000000000000000000 ) ) ;
#1719=ORIENTED_EDGE ( 'NONE', *, *, #112, .F. ) ;
#1720=CARTESIAN_POINT ( 'NONE',  ( 34.73715154119699378, -48.72433491194829713, -2.732636121790667172 ) ) ;
#1726=ORIENTED_EDGE ( 'NONE', *, *, #5264, .F. ) ;
#1727=CARTESIAN_POINT ( 'NONE',  ( 18.03113812440135888, -82.24929059928629727, -4.472107801411128847 ) ) ;
#1732=CARTESIAN_POINT ( 'NONE',  ( 11.74003636399016237, -52.28415370497031489, 3.028416065278661584 ) ) ;
#1736=CARTESIAN_POINT ( 'NONE',  ( 9.358332060254376472, -60.82697974174657674, 1.965378744862418925 ) ) ;
#1738=EDGE_CURVE ( 'NONE', #1089, #9843, #11730, .T. ) ;
#1743=EDGE_LOOP ( 'NONE', ( #3668, #8719, #14872, #8238 ) ) ;
#1755=CARTESIAN_POINT ( 'NONE',  ( 25.17145219045128712, -52.24929059928630437, 4.731961142181925872 ) ) ;
#1763=EDGE_LOOP ( 'NONE', ( #8003, #5857, #4349, #10040 ) ) ;
#1777=CARTESIAN_POINT ( 'NONE',  ( 12.96675353036082257, -65.20845675887582615, -3.989712384465763595 ) ) ;
#1780=CARTESIAN_POINT ( 'NONE',  ( 33.58103295469781813, -55.84923954203684104, 1.895000442030748022 ) ) ;
#1785=CARTESIAN_POINT ( 'NONE',  ( 30.27115683117171585, -61.78784708351293631, -3.496562482608110312 ) ) ;
#1791=CARTESIAN_POINT ( 'NONE',  ( 8.782534692662792963, -56.07151166541877529, 2.830535587930131936 ) ) ;
#1799=ORIENTED_EDGE ( 'NONE', *, *, #5428, .F. ) ;
#1801=CARTESIAN_POINT ( 'NONE',  ( 23.78962786808486740, -62.59345883563879909, -6.358786672826048481 ) ) ;
#1810=EDGE_CURVE ( 'NONE', #304, #9073, #3789, .T. ) ;
#1811=CARTESIAN_POINT ( 'NONE',  ( 12.23810814295288019, -62.76259148841472069, 3.786770376139185323 ) ) ;
#1817=CARTESIAN_POINT ( 'NONE',  ( 8.875263511806062766, -60.06858080083353002, 1.862453320361853182 ) ) ;
#1819=DIRECTION ( 'NONE',  ( -0.9421718071228326608, -7.134436752378406426E-17, 0.3351302520855077849 ) ) ;
#1826=ORIENTED_EDGE ( 'NONE', *, *, #7252, .T. ) ;
#1828=VERTEX_POINT ( 'NONE', #333 ) ;
#1839=CARTESIAN_POINT ( 'NONE',  ( 8.599030766203954457, -59.21224831720009973, -1.832439066040443043 ) ) ;
#1847=CARTESIAN_POINT ( 'NONE',  ( 12.41997800841440913, -64.16417350152465815, -3.791131921652696857 ) ) ;
#1851=ORIENTED_EDGE ( 'NONE', *, *, #1518, .T. ) ;
#1852=CARTESIAN_POINT ( 'NONE',  ( 30.84974339222601003, -61.21674351969437566, -3.284692946547116854 ) ) ;
#1857=CARTESIAN_POINT ( 'NONE',  ( 8.902849800389361690, -55.58404325705457438, 2.908775817946469111 ) ) ;
#1858=EDGE_CURVE ( 'NONE', #14011, #8692, #13111, .T. ) ;
#1861=CARTESIAN_POINT ( 'NONE',  ( 31.72322230991231962, -61.42570632716525125, -2.132522520905369312 ) ) ;
#1864=CARTESIAN_POINT ( 'NONE',  ( 28.59326752685518258, -57.14688517103346044, -4.208364645982451968 ) ) ;
#1869=ORIENTED_EDGE ( 'NONE', *, *, #4253, .T. ) ;
#1874=CARTESIAN_POINT ( 'NONE',  ( 13.15370223272280370, -65.65107448351760411, 3.408697305258708621 ) ) ;
#1885=DIRECTION ( 'NONE',  ( -0.000000000000000000, -0.000000000000000000, -1.000000000000000000 ) ) ;
#1891=CIRCLE ( 'NONE', #11736, 0.9999999999999993339 ) ;
#1892=CYLINDRICAL_SURFACE ( 'NONE', #13333, 3.999999999999999112 ) ;
#1913=EDGE_CURVE ( 'NONE', #12651, #13625, #1487, .T. ) ;
#1914=CARTESIAN_POINT ( 'NONE',  ( 27.33382790127958728, -69.39711819508849544, 4.502057496415716287 ) ) ;
#1923=CARTESIAN_POINT ( 'NONE',  ( 11.75462132594792131, -63.18892729117400364, -3.546101824478771203 ) ) ;
#1929=CARTESIAN_POINT ( 'NONE',  ( 31.49298359385885959, -60.71197230342421136, -3.050751728647420613 ) ) ;
#1934=CARTESIAN_POINT ( 'NONE',  ( 11.55337909437054478, -53.31401535610196163, 3.970404413101017216 ) ) ;
#1935=CARTESIAN_POINT ( 'NONE',  ( 13.77203033081066330, -67.83931925369921601, 3.638954064322520665 ) ) ;
#1942=CARTESIAN_POINT ( 'NONE',  ( 31.74929939486185404, -60.51083307721700777, 2.957531760941162435 ) ) ;
#1944=CARTESIAN_POINT ( 'NONE',  ( 27.25618691382818781, -52.24929059928630437, -3.946674196986641903 ) ) ;
#1945=CARTESIAN_POINT ( 'NONE',  ( 8.317129627286451665, -55.12654146333685645, 1.982842638417584791 ) ) ;
#1951=CARTESIAN_POINT ( 'NONE',  ( 13.92771027672793061, -66.12098470289663510, 4.407543342774133066 ) ) ;
#1953=CARTESIAN_POINT ( 'NONE',  ( 10.16048094673748459, -52.84914412566558894, 3.506280953151645896 ) ) ;
#1959=ORIENTED_EDGE ( 'NONE', *, *, #12909, .T. ) ;
#1960=CARTESIAN_POINT ( 'NONE',  ( 13.81529256454321519, -67.42878071148635399, -4.083908651492614617 ) ) ;
#1962=CARTESIAN_POINT ( 'NONE',  ( 32.37487573296866117, -54.69456399997503127, -3.125517714509074452 ) ) ;
#1964=CARTESIAN_POINT ( 'NONE',  ( 28.20373290646733722, -66.75404937493291868, 3.551013195539360012 ) ) ;
#1967=CARTESIAN_POINT ( 'NONE',  ( 20.86173033120691045, -52.24929059928630437, 0.000000000000000000 ) ) ;
#1968=EDGE_CURVE ( 'NONE', #5446, #15191, #10679, .T. ) ;
#1973=CARTESIAN_POINT ( 'NONE',  ( 18.24487436548682240, -53.24929059928630437, 6.492462156583986399 ) ) ;
#1974=CARTESIAN_POINT ( 'NONE',  ( 8.871493660177725005, -54.05847863454847158, -2.186919301701681473 ) ) ;
#1976=CARTESIAN_POINT ( 'NONE',  ( 33.38971411695204949, -58.06117555224668081, 1.821720187977000638 ) ) ;
#1977=ADVANCED_FACE ( 'NONE', ( #4185 ), #5430, .F. ) ;
#1988=CARTESIAN_POINT ( 'NONE',  ( 10.23047706855410688, -60.71197230342353635, -3.050751728647111083 ) ) ;
#1993=CARTESIAN_POINT ( 'NONE',  ( 20.86173033120691045, -52.24929059928630437, 0.000000000000000000 ) ) ;
#1994=CARTESIAN_POINT ( 'NONE',  ( 14.38963276113423895, -69.39711819508849544, 4.502057496415707405 ) ) ;
#1997=FACE_OUTER_BOUND ( 'NONE', #3421, .T. ) ;
#2003=VECTOR ( 'NONE', #9083, 1000.000000000000000 ) ;
#2010=ORIENTED_EDGE ( 'NONE', *, *, #882, .F. ) ;
#2018=DIRECTION ( 'NONE',  ( 0.000000000000000000, 0.000000000000000000, -1.000000000000000000 ) ) ;
#2034=CARTESIAN_POINT ( 'NONE',  ( 13.41074896738031264, -66.37912134691028143, 3.509717431434834722 ) ) ;
#2041=PRODUCT_DEFINITION_SHAPE ( 'NONE', 'NONE',  #6372 ) ;
#2043=DIRECTION ( 'NONE',  ( -0.9744556954135530358, 0.2245798247307378148, 0.000000000000000000 ) ) ;
#2047=CARTESIAN_POINT ( 'NONE',  ( 13.85081399190160667, -68.05329818779055984, -4.069437921243382661 ) ) ;
#2052=CARTESIAN_POINT ( 'NONE',  ( 17.75919831123052361, -66.70789582472772850, -6.276998965480669490 ) ) ;
#2056=AXIS2_PLACEMENT_3D ( 'NONE', #14986, #11355, #816 ) ;
#2061=CARTESIAN_POINT ( 'NONE',  ( 8.696318251036124991, -54.32767344845774460, -2.126657344578855025 ) ) ;
#2062=CARTESIAN_POINT ( 'NONE',  ( 17.09549820959326638, -96.56299909827106376, 1.347403282660979640 ) ) ;
#2063=EDGE_CURVE ( 'NONE', #7033, #5832, #2905, .T. ) ;
#2064=CARTESIAN_POINT ( 'NONE',  ( 20.86173033120691045, -82.24929059928629727, 0.000000000000000000 ) ) ;
#2076=CARTESIAN_POINT ( 'NONE',  ( 21.74884261173415467, -85.24929059928631148, -4.000000000000000888 ) ) ;
#2079=CARTESIAN_POINT ( 'NONE',  ( 23.62269406303978769, -57.98711502980034282, 6.432599168432319381 ) ) ;
#2101=CARTESIAN_POINT ( 'NONE',  ( 8.201103799357262858, -57.48563641131178770, -1.816685854991388238 ) ) ;
#2111=CARTESIAN_POINT ( 'NONE',  ( 29.67303256468918704, -52.24929059928631858, -3.113412445639874182 ) ) ;
#2113=FACE_OUTER_BOUND ( 'NONE', #14298, .T. ) ;
#2116=CARTESIAN_POINT ( 'NONE',  ( 7.330417041869147887, -50.37435811144442255, -2.733270617041293260 ) ) ;
#2118=CARTESIAN_POINT ( 'NONE',  ( 32.98173233368826374, -56.83124152802057694, -2.758380730586864171 ) ) ;
#2128=CIRCLE ( 'NONE', #6795, 7.000000000000000000 ) ;
#2131=ORIENTED_EDGE ( 'NONE', *, *, #4198, .T. ) ;
#2135=CARTESIAN_POINT ( 'NONE',  ( 10.22565734178488839, -53.83453582474933086, -3.481203917140358151 ) ) ;
#2136=LINE ( 'NONE', #10378, #6711 ) ;
#2139=FACE_OUTER_BOUND ( 'NONE', #1763, .T. ) ;
#2146=CARTESIAN_POINT ( 'NONE',  ( 8.876893811795392608, -60.07159297390013108, -1.862767969487477027 ) ) ;
#2156=CARTESIAN_POINT ( 'NONE',  ( 33.74050986731716506, -53.52517728502748184, 2.732533236848883718 ) ) ;
#2161=EDGE_CURVE ( 'NONE', #625, #5948, #13973, .T. ) ;
#2162=CARTESIAN_POINT ( 'NONE',  ( 18.61871093201826355, -52.24929059928630437, 5.564967562786263144 ) ) ;
#2169=CARTESIAN_POINT ( 'NONE',  ( 53.81626139532630759, -96.56299909827106376, 11.78977872328355048 ) ) ;
#2177=CARTESIAN_POINT ( 'NONE',  ( 10.58727470799617087, -61.88944072237683969, 2.366779157396520006 ) ) ;
#2183=CARTESIAN_POINT ( 'NONE',  ( 33.12442989620986822, -59.21224831720009973, 1.832439066040439490 ) ) ;
#2192=CARTESIAN_POINT ( 'NONE',  ( 14.40311142432125990, -68.64054039872965518, 4.542265185091991064 ) ) ;
#2208=CARTESIAN_POINT ( 'NONE',  ( 10.87361627771599260, -61.21666426766272906, -3.284656216408360585 ) ) ;
#2211=CARTESIAN_POINT ( 'NONE',  ( 19.97461805067967333, -85.24929059928631148, 6.000000000000001776 ) ) ;
#2214=CARTESIAN_POINT ( 'NONE',  ( 9.625495281565598304, -53.24070755262478372, -2.425727701579292628 ) ) ;
#2220=DIRECTION ( 'NONE',  ( -0.000000000000000000, -1.000000000000000000, -0.000000000000000000 ) ) ;
#2223=ORIENTED_EDGE ( 'NONE', *, *, #13272, .F. ) ;
#2228=ORIENTED_EDGE ( 'NONE', *, *, #1236, .F. ) ;
#2251=CARTESIAN_POINT ( 'NONE',  ( 9.826335989509445312, -61.28833066657258399, 2.085332803602911067 ) ) ;
#2257=ORIENTED_EDGE ( 'NONE', *, *, #8938, .T. ) ;
#2262=CARTESIAN_POINT ( 'NONE',  ( 10.24650954764479494, -52.80227938113591790, 2.609359049418192633 ) ) ;
#2269=AXIS2_PLACEMENT_3D ( 'NONE', #2169, #7871, #5641 ) ;
#2278=AXIS2_PLACEMENT_3D ( 'NONE', #7930, #9165, #11445 ) ;
#2281=CARTESIAN_POINT ( 'NONE',  ( 18.19235006501570240, -55.08889408817020694, -6.471126372656766712 ) ) ;
#2291=CARTESIAN_POINT ( 'NONE',  ( 10.00023835250150483, -61.42570632716525125, -2.132522520905374197 ) ) ;
#2297=CARTESIAN_POINT ( 'NONE',  ( 11.74410493734513494, -52.28363178956084312, -3.029531835798758621 ) ) ;
#2298=PLANE ( 'NONE',  #7952 ) ;
#2301=ORIENTED_EDGE ( 'NONE', *, *, #9727, .T. ) ;
#2302=CARTESIAN_POINT ( 'NONE',  ( 33.39134818683421457, -58.05408529505576354, 2.501672671502764178 ) ) ;
#2304=CARTESIAN_POINT ( 'NONE',  ( 9.200644618036296407, -59.06479067038043240, -2.757123406423053424 ) ) ;
#2309=FACE_OUTER_BOUND ( 'NONE', #14743, .T. ) ;
#2318=CARTESIAN_POINT ( 'NONE',  ( 32.86365436560006259, -57.78392871903673012, 2.727962224263459134 ) ) ;
#2336=VERTEX_POINT ( 'NONE', #1994 ) ;
#2337=ORIENTED_EDGE ( 'NONE', *, *, #2161, .T. ) ;
#2339=B_SPLINE_CURVE_WITH_KNOTS ( 'NONE', 3,
 ( #5211, #9916, #14594, #8738, #7748, #10209, #12516, #4271, #14742, #1962, #5438, #3056, #12433, #7900, #7980, #2118, #3356, #5675 ),
 .UNSPECIFIED., .F., .F.,
 ( 4, 2, 2, 2, 2, 2, 2, 2, 4 ),
 ( 8.673617379884035472E-19, 0.0007600084067931453437, 0.001520016813586290471, 0.002280025220379426707, 0.003040033627172562727, 0.003800042033965699180, 0.004560050440758835200, 0.005320058847551972087, 0.006080067254345108106 ),
 .UNSPECIFIED. ) ;
#2341=CARTESIAN_POINT ( 'NONE',  ( 12.36791015745245836, -52.24929059928631148, -3.199931146564426232 ) ) ;
#2342=CARTESIAN_POINT ( 'NONE',  ( 23.47858629692699139, -53.24929059928630437, 6.492462156583989064 ) ) ;
#2345=CARTESIAN_POINT ( 'NONE',  ( 8.201103799357262858, -57.48563641131178770, 2.500000000000000000 ) ) ;
#2351=CARTESIAN_POINT ( 'NONE',  ( 33.02714241137783802, -54.32767344845796487, 2.126657344578741338 ) ) ;
#2368=EDGE_CURVE ( 'NONE', #625, #7109, #1514, .T. ) ;
#2377=CARTESIAN_POINT ( 'NONE',  ( 10.87371727018780199, -61.21674351969439698, 3.284692946547135950 ) ) ;
#2378=VERTEX_POINT ( 'NONE', #6020 ) ;
#2390=CIRCLE ( 'NONE', #9018, 31.00000000000000000 ) ;
#2396=EDGE_CURVE ( 'NONE', #13625, #4027, #14883, .T. ) ;
#2397=CIRCLE ( 'NONE', #651, 1.000000000000000888 ) ;
#2400=DIRECTION ( 'NONE',  ( 0.000000000000000000, 1.000000000000000000, 0.000000000000000000 ) ) ;
#2407=CARTESIAN_POINT ( 'NONE',  ( 32.32366773688528383, -59.70501925844574487, -2.784164790581364457 ) ) ;
#2410=VECTOR ( 'NONE', #3998, 1000.000000000000000 ) ;
#2412=CARTESIAN_POINT ( 'NONE',  ( 28.80923764261828524, -63.78832907041062583, 4.037694147267533396 ) ) ;
#2414=CARTESIAN_POINT ( 'NONE',  ( 32.28540069953670866, -53.39764053564380220, -3.230171433733334485 ) ) ;
#2417=ORIENTED_EDGE ( 'NONE', *, *, #13987, .F. ) ;
#2421=CARTESIAN_POINT ( 'NONE',  ( 8.234143183932166821, -55.39494951565961856, -1.945583896730202378 ) ) ;
#2431=CARTESIAN_POINT ( 'NONE',  ( 14.10690393411112531, -69.39711819508849544, 4.282389493064012953 ) ) ;
#2432=CARTESIAN_POINT ( 'NONE',  ( 32.87864669132871143, -54.08909618700784705, 2.984935890592543828 ) ) ;
#2434=FACE_OUTER_BOUND ( 'NONE', #4508, .T. ) ;
#2444=CARTESIAN_POINT ( 'NONE',  ( 8.121007193492978615, -55.93345933723870900, 2.599599694947450246 ) ) ;
#2446=CARTESIAN_POINT ( 'NONE',  ( 19.97461805067967333, -82.24929059928629727, 6.000000000000001776 ) ) ;
#2450=AXIS2_PLACEMENT_3D ( 'NONE', #9013, #15022, #3321 ) ;
#2456=CARTESIAN_POINT ( 'NONE',  ( 28.56975842969000823, -65.65107448352046049, 3.408697305255369514 ) ) ;
#2457=ORIENTED_EDGE ( 'NONE', *, *, #4253, .F. ) ;
#2486=CARTESIAN_POINT ( 'NONE',  ( 29.35555050496135010, -52.24929059928631148, -3.199931146564412909 ) ) ;
#2507=FACE_OUTER_BOUND ( 'NONE', #6371, .T. ) ;
#2508=ORIENTED_EDGE ( 'NONE', *, *, #7909, .F. ) ;
#2509=DIRECTION ( 'NONE',  ( 0.000000000000000000, -0.000000000000000000, 1.000000000000000000 ) ) ;
#2511=APPLICATION_CONTEXT ( 'automotive_design' ) ;
#2517=VERTEX_POINT ( 'NONE', #6249 ) ;
#2522=CARTESIAN_POINT ( 'NONE',  ( 13.41466460742226019, -66.31562986446989783, -3.513916789801494911 ) ) ;
#2524=CARTESIAN_POINT ( 'NONE',  ( 8.741768373587657237, -56.83327624868845618, 2.758240060640735791 ) ) ;
#2534=CARTESIAN_POINT ( 'NONE',  ( 9.488565264687794709, -59.84608319322163794, -2.809346289342996794 ) ) ;
#2536=CARTESIAN_POINT ( 'NONE',  ( 20.86173033120691045, -72.24929059928631148, -3.999999999999999112 ) ) ;
#2548=( BOUNDED_SURFACE ( )  B_SPLINE_SURFACE ( 3, 2, ( 
 ( #12668, #13819, #9212 ),
 ( #5673, #1112, #13744 ),
 ( #4584, #3281, #2281 ),
 ( #2116, #9362, #10520 ),
 ( #808, #15133, #13899 ),
 ( #7897, #10289, #15208 ),
 ( #8054, #6892, #10361 ),
 ( #15059, #3199, #12512 ),
 ( #9287, #4664, #3353 ),
 ( #14055, #4509, #880 ),
 ( #13979, #10205, #7827 ),
 ( #1044, #1960, #5595 ),
 ( #6656, #2047, #11347 ),
 ( #11582, #5520, #4348 ) ),
 .UNSPECIFIED., .F., .F., .F. ) 
 B_SPLINE_SURFACE_WITH_KNOTS ( ( 4, 2, 2, 2, 2, 2, 4 ),
 ( 3, 3 ),
 ( 0.2948322565876038137, 0.2981287057529115603, 0.3014251549182193068, 0.3080180532488348000, 0.3146109515794502931, 0.3179074007447579842, 0.3212038499100657307 ),
 ( 0.07447800286616054755, 1.000000000000000000 ),
 .UNSPECIFIED. ) 
 GEOMETRIC_REPRESENTATION_ITEM ( )  RATIONAL_B_SPLINE_SURFACE ( (
 ( 0.9996905063672956171, 0.9979222480410725460, 1.000000000000000000),
 ( 0.9996957508213744070, 0.9979574561151137724, 1.000000000000000000),
 ( 0.9997005874846982554, 0.9979899265301206412, 1.000000000000000000),
 ( 0.9997092625818566614, 0.9980481658546502821, 1.000000000000000000),
 ( 0.9997131045178146991, 0.9980739582752989891, 1.000000000000000000),
 ( 0.9997231512649209506, 0.9981414060230869856, 1.000000000000000000),
 ( 0.9997278760137982001, 0.9981731251125871562, 1.000000000000000000),
 ( 0.9997334421747965383, 0.9982104929311652608, 1.000000000000000000),
 ( 0.9997342833619657920, 0.9982161401500547759, 1.000000000000000000),
 ( 0.9997327054743884167, 0.9982055471728220608, 1.000000000000000000),
 ( 0.9997317056072283492, 0.9981988346730122919, 1.000000000000000000),
 ( 0.9997287795965361656, 0.9981791912173640924, 1.000000000000000000),
 ( 0.9997268671536080342, 0.9981663522390450405, 1.000000000000000000),
 ( 0.9997245403443033585, 0.9981507314569679767, 1.000000000000000000) ) ) 
 REPRESENTATION_ITEM ( '' )  SURFACE ( )  );
#2560=ORIENTED_EDGE ( 'NONE', *, *, #9418, .T. ) ;
#2565=CARTESIAN_POINT ( 'NONE',  ( 18.22133905412741228, -54.09900330348943953, 6.482993899721375186 ) ) ;
#2566=DIRECTION ( 'NONE',  ( -0.000000000000000000, 1.000000000000000000, -0.000000000000000000 ) ) ;
#2570=CARTESIAN_POINT ( 'NONE',  ( 30.00467404504382785, -52.27436801239488062, -4.068677752280153825 ) ) ;
#2583=CARTESIAN_POINT ( 'NONE',  ( 32.96267541773152487, -54.21582538152092212, 2.947777686198818081 ) ) ;
#2588=ORIENTED_EDGE ( 'NONE', *, *, #11320, .T. ) ;
#2594=CARTESIAN_POINT ( 'NONE',  ( 8.216359860972971774, -55.48278564389666911, 2.668166895090217761 ) ) ;
#2605=CARTESIAN_POINT ( 'NONE',  ( 29.73572575534515749, -63.50313342087166291, 3.632148419033245812 ) ) ;
#2614=AXIS2_PLACEMENT_3D ( 'NONE', #11749, #10212, #6899 ) ;
#2619=ADVANCED_FACE ( 'NONE', ( #8685 ), #4134, .T. ) ;
#2622=CARTESIAN_POINT ( 'NONE',  ( 32.48948299040029042, -60.63235088943246609, -1.938839523630887074 ) ) ;
#2630=SHAPE_REPRESENTATION ( 'Plastic-Headed Clamping Screw', ( #6315 ), #5577 ) ;
#2632=CARTESIAN_POINT ( 'NONE',  ( 8.286643821053985448, -55.00297582946176789, 2.730999879045922896 ) ) ;
#2639=CARTESIAN_POINT ( 'NONE',  ( 31.29089880224823617, -53.71411213207086632, -3.559347964322167268 ) ) ;
#2642=EDGE_LOOP ( 'NONE', ( #14948, #6854, #1726, #4839 ) ) ;
#2644=CARTESIAN_POINT ( 'NONE',  ( 32.23491518596268435, -59.84602720838576317, -2.809343037843366364 ) ) ;
#2647=CARTESIAN_POINT ( 'NONE',  ( 20.86173033120691045, -53.24929059928630437, 0.000000000000000000 ) ) ;
#2658=CARTESIAN_POINT ( 'NONE',  ( 30.30473640079415887, -52.33170319195768627, 3.962365649672984880 ) ) ;
#2663=CARTESIAN_POINT ( 'NONE',  ( 53.81626139532630049, -85.24929059928631148, -11.78977872328356646 ) ) ;
#2669=ORIENTED_EDGE ( 'NONE', *, *, #10456, .F. ) ;
#2681=CARTESIAN_POINT ( 'NONE',  ( 29.65531183511369662, -63.62021712492886394, 2.966460067269240497 ) ) ;
#2683=CARTESIAN_POINT ( 'NONE',  ( 23.69232253801246202, -96.56299909827106376, 4.472107801411124406 ) ) ;
#2684=LINE ( 'NONE', #5071, #5469 ) ;
#2686=CARTESIAN_POINT ( 'NONE',  ( 28.75670713205333229, -65.20845675887589721, -3.989712384466157058 ) ) ;
#2689=ADVANCED_FACE ( 'NONE', ( #598 ), #10910, .T. ) ;
#2691=AXIS2_PLACEMENT_3D ( 'NONE', #10185, #13721, #2018 ) ;
#2699=ORIENTED_EDGE ( 'NONE', *, *, #5308, .F. ) ;
#2710=CARTESIAN_POINT ( 'NONE',  ( 18.19235006502503893, -55.08889408817012168, 6.471126372660669368 ) ) ;
#2712=CARTESIAN_POINT ( 'NONE',  ( 29.67377849276340385, -52.24929059928631148, 3.113209168868824595 ) ) ;
#2714=CARTESIAN_POINT ( 'NONE',  ( 30.85841852505513572, -53.50006564588471036, -3.720697674323108828 ) ) ;
#2716=EDGE_LOOP ( 'NONE', ( #102, #13483, #13190, #13571 ) ) ;
#2717=CARTESIAN_POINT ( 'NONE',  ( 8.091875466796944139, -56.52532528994184702, -1.842181053809134994 ) ) ;
#2726=ORIENTED_EDGE ( 'NONE', *, *, #6143, .T. ) ;
#2728=CARTESIAN_POINT ( 'NONE',  ( 34.91294709002737306, -47.87885576610680971, -2.732387392806885806 ) ) ;
#2734=ORIENTED_EDGE ( 'NONE', *, *, #1130, .F. ) ;
#2739=EDGE_CURVE ( 'NONE', #10002, #9843, #3218, .T. ) ;
#2754=EDGE_CURVE ( 'NONE', #10773, #4753, #11577, .T. ) ;
#2756=VERTEX_POINT ( 'NONE', #1036 ) ;
#2758=CARTESIAN_POINT ( 'NONE',  ( 29.35555050496136431, -53.24929059928631148, 3.199931146564425788 ) ) ;
#2760=CARTESIAN_POINT ( 'NONE',  ( 28.23010146221949768, -64.93526722763043324, 4.251815205946187781 ) ) ;
#2761=ORIENTED_EDGE ( 'NONE', *, *, #6621, .F. ) ;
#2768=CARTESIAN_POINT ( 'NONE',  ( 28.33202942550260417, -66.31583591551820689, -4.137138225905601985 ) ) ;
#2780=CIRCLE ( 'NONE', #12865, 1.000000000000001332 ) ;
#2787=CARTESIAN_POINT ( 'NONE',  ( 7.328728967433968400, -50.37334675436643749, 2.732818608233515079 ) ) ;
#2791=CARTESIAN_POINT ( 'NONE',  ( 32.46725937536812268, -53.58811172139414936, 2.311880426527626486 ) ) ;
#2792=CARTESIAN_POINT ( 'NONE',  ( 14.31939787081870286, -67.79239290436674992, -4.531617596073229670 ) ) ;
#2803=CARTESIAN_POINT ( 'NONE',  ( 12.03298173962126683, -53.28399145779480506, 4.141535524925028078 ) ) ;
#2807=CARTESIAN_POINT ( 'NONE',  ( 8.464703746082088642, -58.62940108252796279, -2.501915095525329757 ) ) ;
#2811=CARTESIAN_POINT ( 'NONE',  ( 18.61871093201826000, -52.24929059928630437, 5.564967562786272914 ) ) ;
#2817=CARTESIAN_POINT ( 'NONE',  ( 11.08978525922602465, -53.42148821037783790, 3.802824752091033211 ) ) ;
#2823=FACE_OUTER_BOUND ( 'NONE', #6199, .T. ) ;
#2825=FACE_OUTER_BOUND ( 'NONE', #8689, .T. ) ;
#2848=CARTESIAN_POINT ( 'NONE',  ( 8.858401005300839515, -57.78267463917103441, 2.727521282215370935 ) ) ;
#2855=CIRCLE ( 'NONE', #12962, 7.000000000000000000 ) ;
#2858=CARTESIAN_POINT ( 'NONE',  ( 20.86173033120691045, -82.24929059928629727, 0.000000000000000000 ) ) ;
#2859=CARTESIAN_POINT ( 'NONE',  ( 8.201103799357262858, -57.48563641131178770, -1.816685854991388238 ) ) ;
#2864=CIRCLE ( 'NONE', #4845, 3.000000000000000888 ) ;
#2871=TOROIDAL_SURFACE ( 'NONE', #3365, 6.000000000000000000, 1.000000000000000000 ) ;
#2875=AXIS2_PLACEMENT_3D ( 'NONE', #1034, #14047, #14970 ) ;
#2882=CARTESIAN_POINT ( 'NONE',  ( 13.95756414556647762, -69.39711819508849544, -4.056575093033447210 ) ) ;
#2888=CARTESIAN_POINT ( 'NONE',  ( 11.71878661736996108, -52.27436801240079944, 4.068677752283970328 ) ) ;
#2896=CARTESIAN_POINT ( 'NONE',  ( 10.00023835250150483, -61.42570632716525125, 2.132522520905368868 ) ) ;
#2905=CIRCLE ( 'NONE', #12002, 7.000000000000000000 ) ;
#2907=CARTESIAN_POINT ( 'NONE',  ( 20.86173033120691045, -72.24929059928631148, 7.000000000000000000 ) ) ;
#2909=CARTESIAN_POINT ( 'NONE',  ( 29.30348265399867103, -64.16417350152767085, -3.791131921649141034 ) ) ;
#2911=B_SPLINE_CURVE_WITH_KNOTS ( 'NONE', 3,
 ( #239, #8544, #1542, #8399 ),
 .UNSPECIFIED., .F., .F.,
 ( 4, 4 ),
 ( 0.000000000000000000, 0.003645914952990591488 ),
 .UNSPECIFIED. ) ;
#2912=CARTESIAN_POINT ( 'NONE',  ( 27.25620696618382865, -52.24929059928630437, 3.946667064627068733 ) ) ;
#2922=VERTEX_POINT ( 'NONE', #1109 ) ;
#2928=DIRECTION ( 'NONE',  ( 0.000000000000000000, -0.000000000000000000, 1.000000000000000000 ) ) ;
#2937=CARTESIAN_POINT ( 'NONE',  ( 10.00023835250150128, -61.42570632716525125, -2.132522520905388852 ) ) ;
#2948=( NAMED_UNIT ( * ) SI_UNIT ( $, .STERADIAN. ) SOLID_ANGLE_UNIT ( ) );
#2959=CARTESIAN_POINT ( 'NONE',  ( 34.39473169496078242, -50.37334675433798026, -2.732818608182232989 ) ) ;
#2972=CARTESIAN_POINT ( 'NONE',  ( 12.02094163398139948, -52.24929059928630437, 4.175384597093459327 ) ) ;
#2985=EDGE_CURVE ( 'NONE', #4765, #3836, #11556, .T. ) ;
#2987=ORIENTED_EDGE ( 'NONE', *, *, #5655, .T. ) ;
#2989=DIRECTION ( 'NONE',  ( 0.000000000000000000, 0.000000000000000000, 1.000000000000000000 ) ) ;
#2995=CARTESIAN_POINT ( 'NONE',  ( 12.03298173962126327, -53.28399145779480506, -4.141535524925033407 ) ) ;
#3002=AXIS2_PLACEMENT_3D ( 'NONE', #14403, #13102, #10865 ) ;
#3007=CARTESIAN_POINT ( 'NONE',  ( 20.86173033120691045, -52.24929059928630437, 3.000000000000000888 ) ) ;
#3016=DIRECTION ( 'NONE',  ( 0.000000000000000000, -1.000000000000000000, 0.000000000000000000 ) ) ;
#3019=CARTESIAN_POINT ( 'NONE',  ( 33.63076355350840174, -56.34136508318270842, 1.853100783822632325 ) ) ;
#3025=FACE_OUTER_BOUND ( 'NONE', #3144, .T. ) ;
#3028=CARTESIAN_POINT ( 'NONE',  ( 11.79087746573607909, -53.28557432868839072, 4.055360768046006648 ) ) ;
#3035=CARTESIAN_POINT ( 'NONE',  ( 27.95143033160315582, -67.83931925369921601, -3.638954064322521553 ) ) ;
#3041=CARTESIAN_POINT ( 'NONE',  ( 29.35555050496136786, -52.24929059928630437, -3.199931146564429341 ) ) ;
#3045=CARTESIAN_POINT ( 'NONE',  ( 13.87384783255121690, -69.39711819508849544, -3.799217554615847980 ) ) ;
#3046=CARTESIAN_POINT ( 'NONE',  ( 12.66974950169162284, -64.60713873539378937, 3.212402267261584399 ) ) ;
#3053=CARTESIAN_POINT ( 'NONE',  ( 9.200644618036292854, -59.06479067038041819, 2.757123406423321210 ) ) ;
#3054=EDGE_CURVE ( 'NONE', #4027, #143, #12657, .T. ) ;
#3056=CARTESIAN_POINT ( 'NONE',  ( 32.73440452410881107, -55.35059346084329235, -2.955710789589959919 ) ) ;
#3057=ORIENTED_EDGE ( 'NONE', *, *, #7991, .T. ) ;
#3058=CARTESIAN_POINT ( 'NONE',  ( 27.94158133900394958, -67.90279320103996952, 3.641642753168639501 ) ) ;
#3067=DIRECTION ( 'NONE',  ( -0.000000000000000000, 1.000000000000000000, -0.000000000000000000 ) ) ;
#3080=ADVANCED_FACE ( 'NONE', ( #13639 ), #8950, .F. ) ;
#3083=CARTESIAN_POINT ( 'NONE',  ( 18.24487436548682950, -53.24929059928630437, -6.492462156583989064 ) ) ;
#3084=CARTESIAN_POINT ( 'NONE',  ( 11.98773490706720324, -63.50313342087172686, -3.632148419031555608 ) ) ;
#3089=CARTESIAN_POINT ( 'NONE',  ( 13.86173033120691223, -69.39711819508849544, -3.619682905202625811 ) ) ;
#3094=CARTESIAN_POINT ( 'NONE',  ( 10.21747785520277851, -53.84004999663768132, 3.478067438360142205 ) ) ;
#3097=DIRECTION ( 'NONE',  ( -0.000000000000000000, 1.000000000000000000, -0.000000000000000000 ) ) ;
#3103=CARTESIAN_POINT ( 'NONE',  ( 25.53134746123848231, -53.25924031079294707, -5.665074923594188405 ) ) ;
#3109=CARTESIAN_POINT ( 'NONE',  ( 20.86173033120691045, -53.24929059928630437, 0.000000000000000000 ) ) ;
#3113=CARTESIAN_POINT ( 'NONE',  ( 13.39143123690971571, -66.31583591551516577, 4.137138225902095456 ) ) ;
#3115=EDGE_CURVE ( 'NONE', #8264, #1089, #6071, .T. ) ;
#3116=CARTESIAN_POINT ( 'NONE',  ( 10.22665806587732362, -53.84195147944168269, 3.481029309661981319 ) ) ;
#3117=CARTESIAN_POINT ( 'NONE',  ( 29.99044527668438320, -52.28496698959959588, -3.026492948547165440 ) ) ;
#3129=CIRCLE ( 'NONE', #9545, 31.00000000000000000 ) ;
#3134=ADVANCED_FACE ( 'NONE', ( #6634 ), #11319, .T. ) ;
#3139=CARTESIAN_POINT ( 'NONE',  ( 9.328516978903417467, -53.50439862579597161, -3.186601206343369075 ) ) ;
#3144=EDGE_LOOP ( 'NONE', ( #11058, #5212, #9723, #10671 ) ) ;
#3151=CARTESIAN_POINT ( 'NONE',  ( 9.755347871979424212, -60.26979819505855573, -2.885043711493008090 ) ) ;
#3154=EDGE_CURVE ( 'NONE', #8543, #12651, #5323, .T. ) ;
#3171=CARTESIAN_POINT ( 'NONE',  ( 27.33382790127957662, -69.39711819508849544, -4.502057496415715399 ) ) ;
#3179=ORIENTED_EDGE ( 'NONE', *, *, #9295, .F. ) ;
#3182=CARTESIAN_POINT ( 'NONE',  ( 20.86173033120691045, -57.24929059928630437, 0.000000000000000000 ) ) ;
#3188=CARTESIAN_POINT ( 'NONE',  ( 9.826704175994500190, -61.28862151863886965, -2.085432713781506742 ) ) ;
#3191=CARTESIAN_POINT ( 'NONE',  ( 32.23489539772602797, -59.84608319322163794, 2.809346289343019443 ) ) ;
#3199=CARTESIAN_POINT ( 'NONE',  ( 13.46836618102747885, -61.89662211388733937, -4.174060188899890278 ) ) ;
#3200=ORIENTED_EDGE ( 'NONE', *, *, #12234, .F. ) ;
#3202=CARTESIAN_POINT ( 'NONE',  ( 32.52281604437752804, -59.06479067038042530, -2.757123406422443690 ) ) ;
#3213=CARTESIAN_POINT ( 'NONE',  ( 8.965898960377726823, -53.92993659400900697, -2.218374547571393851 ) ) ;
#3218=CIRCLE ( 'NONE', #8625, 0.9999999999999993339 ) ;
#3219=CARTESIAN_POINT ( 'NONE',  ( 32.90197589884652274, -57.33450387999030795, 2.749014434309863919 ) ) ;
#3226=PLANE ( 'NONE',  #2278 ) ;
#3228=CARTESIAN_POINT ( 'NONE',  ( 9.347558955408640458, -54.69585338401583385, -3.125080077088496111 ) ) ;
#3231=DIRECTION ( 'NONE',  ( 0.000000000000000000, -0.000000000000000000, 1.000000000000000000 ) ) ;
#3234=CARTESIAN_POINT ( 'NONE',  ( 10.62011700622559829, -60.64100864355887666, 2.132522520905388852 ) ) ;
#3236=ORIENTED_EDGE ( 'NONE', *, *, #1913, .T. ) ;
#3238=CARTESIAN_POINT ( 'NONE',  ( 12.36791015745246014, -53.24929059928630437, -3.199931146564422679 ) ) ;
#3243=VERTEX_POINT ( 'NONE', #3644 ) ;
#3244=CARTESIAN_POINT ( 'NONE',  ( 27.33382790127957662, -69.39711819508849544, -4.502057496415715399 ) ) ;
#3252=CIRCLE ( 'NONE', #7431, 1.000000000000000888 ) ;
#3267=CARTESIAN_POINT ( 'NONE',  ( 9.169527510129993786, -53.67350875049211112, 2.284939533141856494 ) ) ;
#3268=VECTOR ( 'NONE', #14516, 1000.000000000000000 ) ;
#3274=CARTESIAN_POINT ( 'NONE',  ( 32.23803895999753166, -53.36286701831910761, -2.383094873945970971 ) ) ;
#3280=ORIENTED_EDGE ( 'NONE', *, *, #9258, .T. ) ;
#3281=CARTESIAN_POINT ( 'NONE',  ( 12.72586251681365965, -51.89519585600351803, -4.215672594460507128 ) ) ;
#3282=EDGE_LOOP ( 'NONE', ( #4650, #5105, #9693, #11992, #8256, #1503, #1203 ) ) ;
#3294=CARTESIAN_POINT ( 'NONE',  ( 8.171907405451781514, -55.68585955703573376, -1.912302604852146759 ) ) ;
#3296=DIRECTION ( 'NONE',  ( 0.000000000000000000, 0.000000000000000000, -1.000000000000000000 ) ) ;
#3304=CARTESIAN_POINT ( 'NONE',  ( 9.276697446006050285, -60.72048491829438888, -2.646952986712525657 ) ) ;
#3307=CARTESIAN_POINT ( 'NONE',  ( 8.782682478343074806, -56.07092277360308685, -2.830630916608713132 ) ) ;
#3309=EDGE_LOOP ( 'NONE', ( #1351, #5223, #4669, #8233, #9793, #14603, #6056 ) ) ;
#3314=CARTESIAN_POINT ( 'NONE',  ( 25.53134746123851784, -53.25924031079306786, 5.665074923594168865 ) ) ;
#3321=DIRECTION ( 'NONE',  ( 0.000000000000000000, 0.000000000000000000, -1.000000000000000000 ) ) ;
#3325=B_SPLINE_CURVE_WITH_KNOTS ( 'NONE', 3,
 ( #8008, #5789, #10320, #11621 ),
 .UNSPECIFIED., .F., .F.,
 ( 4, 4 ),
 ( 0.000000000000000000, 0.006642668954637878306 ),
 .UNSPECIFIED. ) ;
#3330=CARTESIAN_POINT ( 'NONE',  ( 13.41466460742225308, -66.31562986446988361, 3.513916789801492691 ) ) ;
#3331=CARTESIAN_POINT ( 'NONE',  ( 8.821484763567294607, -57.33450387999030795, 2.749014434309869248 ) ) ;
#3335=CARTESIAN_POINT ( 'NONE',  ( 31.88160194160486327, -62.60511169121411967, -2.715102820263733729 ) ) ;
#3337=CARTESIAN_POINT ( 'NONE',  ( 23.47858629692700205, -52.24929059928630437, -6.492462156583976629 ) ) ;
#3338=CARTESIAN_POINT ( 'NONE',  ( 23.96426235118327597, -66.70789582472760060, 6.276998965480676596 ) ) ;
#3347=CARTESIAN_POINT ( 'NONE',  ( 33.43599298439418277, -55.23669688164211777, -1.968664552513456956 ) ) ;
#3353=CARTESIAN_POINT ( 'NONE',  ( 17.70648456745510657, -67.68160391995883174, -6.249260988559856678 ) ) ;
#3356=CARTESIAN_POINT ( 'NONE',  ( 32.95720782078544886, -57.08298494442341564, -2.747852995220870564 ) ) ;
#3363=CARTESIAN_POINT ( 'NONE',  ( 24.10826840236109803, -69.39711819508849544, -6.201611931792124111 ) ) ;
#3365=AXIS2_PLACEMENT_3D ( 'NONE', #5286, #728, #10986 ) ;
#3370=CARTESIAN_POINT ( 'NONE',  ( 8.344481171119126017, -55.03829860714187561, -2.746682580607167079 ) ) ;
#3374=ORIENTED_EDGE ( 'NONE', *, *, #1518, .F. ) ;
#3378=DIRECTION ( 'NONE',  ( -0.2245716668862467735, 0.9744202983869691970, 0.008523410314123130646 ) ) ;
#3381=AXIS2_PLACEMENT_3D ( 'NONE', #3704, #14337, #12010 ) ;
#3392=CARTESIAN_POINT ( 'NONE',  ( 24.31690506112493111, -73.00063092931685560, 6.088059227055016898 ) ) ;
#3396=ORIENTED_EDGE ( 'NONE', *, *, #13536, .T. ) ;
#3402=CARTESIAN_POINT ( 'NONE',  ( 20.86173033120691045, -72.24929059928631148, 0.000000000000000000 ) ) ;
#3405=ORIENTED_EDGE ( 'NONE', *, *, #13767, .F. ) ;
#3419=CARTESIAN_POINT ( 'NONE',  ( 8.317699921865331802, -55.12535711695123553, -1.983057912332487627 ) ) ;
#3421=EDGE_LOOP ( 'NONE', ( #15097, #14300, #3236, #9525, #6608, #12971, #10003 ) ) ;
#3424=CARTESIAN_POINT ( 'NONE',  ( 8.599030766203958009, -59.21224831720011395, -1.832439066039622144 ) ) ;
#3426=VECTOR ( 'NONE', #12716, 1000.000000000000000 ) ;
#3440=VERTEX_POINT ( 'NONE', #13776 ) ;
#3445=ORIENTED_EDGE ( 'NONE', *, *, #11700, .F. ) ;
#3448=CARTESIAN_POINT ( 'NONE',  ( 9.167911396685996195, -53.68459816487493441, -2.283893849732906656 ) ) ;
#3449=DIRECTION ( 'NONE',  ( 0.000000000000000000, -1.000000000000000000, 0.000000000000000000 ) ) ;
#3457=CARTESIAN_POINT ( 'NONE',  ( 14.30638130925798812, -67.70775585802554986, 4.528449950254405110 ) ) ;
#3472=ORIENTED_EDGE ( 'NONE', *, *, #5951, .F. ) ;
#3480=DIRECTION ( 'NONE',  ( 0.000000000000000000, -1.000000000000000000, 0.000000000000000000 ) ) ;
#3492=ADVANCED_FACE ( 'NONE', ( #11383 ), #14617, .T. ) ;
#3494=AXIS2_PLACEMENT_3D ( 'NONE', #8573, #12181, #484 ) ;
#3498=CARTESIAN_POINT ( 'NONE',  ( 9.786677144408656659, -53.10505385066578299, -2.474491299097422825 ) ) ;
#3499=CARTESIAN_POINT ( 'NONE',  ( 17.75919831123052717, -66.70789582472760060, 6.276998965480673043 ) ) ;
#3508=CARTESIAN_POINT ( 'NONE',  ( 8.201103799357262858, -57.48563641131178770, -1.816685854991388238 ) ) ;
#3515=EDGE_LOOP ( 'NONE', ( #11920, #3534 ) ) ;
#3524=CARTESIAN_POINT ( 'NONE',  ( 18.16985775135672654, -55.94205978621076980, -6.462225911923646926 ) ) ;
#3525=CARTESIAN_POINT ( 'NONE',  ( 11.11753584644738346, -62.41236107492795071, -2.580051240451687988 ) ) ;
#3526=CIRCLE ( 'NONE', #10157, 1.000000000000000222 ) ;
#3534=ORIENTED_EDGE ( 'NONE', *, *, #11664, .T. ) ;
#3536=CARTESIAN_POINT ( 'NONE',  ( 9.984269850081815889, -60.50127194134182673, -2.962969586007857092 ) ) ;
#3542=CARTESIAN_POINT ( 'NONE',  ( 20.86173033120691045, -82.24929059928629727, 3.999999999999999112 ) ) ;
#3545=ADVANCED_FACE ( 'NONE', ( #11236 ), #7841, .T. ) ;
#3546=DIRECTION ( 'NONE',  ( 0.000000000000000000, 1.000000000000000000, 0.000000000000000000 ) ) ;
#3548=FACE_OUTER_BOUND ( 'NONE', #2642, .T. ) ;
#3557=CARTESIAN_POINT ( 'NONE',  ( 27.86173033120691045, -69.39711819508849544, 3.619682905202613377 ) ) ;
#3561=CARTESIAN_POINT ( 'NONE',  ( 32.18160929697071992, -61.03551305047646736, -2.732671606847018264 ) ) ;
#3570=CARTESIAN_POINT ( 'NONE',  ( 8.127390121783262700, -55.95709369454765891, -1.884733065488557902 ) ) ;
#3575=CARTESIAN_POINT ( 'NONE',  ( 14.38836832001927846, -69.49659648540917090, 4.497058153269694714 ) ) ;
#3576=EDGE_CURVE ( 'NONE', #14799, #10038, #7555, .T. ) ;
#3579=DIRECTION ( 'NONE',  ( 0.000000000000000000, 1.000000000000000000, 0.000000000000000000 ) ) ;
#3580=CARTESIAN_POINT ( 'NONE',  ( 33.11767511809988207, -54.47948885957446663, 2.876625435111399121 ) ) ;
#3584=ADVANCED_FACE ( 'NONE', ( #1997 ), #6193, .F. ) ;
#3587=CARTESIAN_POINT ( 'NONE',  ( 12.03298173962126683, -53.28399145779480506, 4.141535524925028078 ) ) ;
#3594=FACE_OUTER_BOUND ( 'NONE', #9135, .T. ) ;
#3595=CARTESIAN_POINT ( 'NONE',  ( 8.753908754604131204, -54.21180406361235526, 2.945963350965704386 ) ) ;
#3596=CARTESIAN_POINT ( 'NONE',  ( 8.821484763567292831, -57.33450387999030795, -2.749014434309867028 ) ) ;
#3597=CARTESIAN_POINT ( 'NONE',  ( 10.00023835250150483, -61.42570632716525125, 2.132522520905371977 ) ) ;
#3604=ORIENTED_EDGE ( 'NONE', *, *, #13833, .F. ) ;
#3605=FACE_OUTER_BOUND ( 'NONE', #10290, .T. ) ;
#3617=ORIENTED_EDGE ( 'NONE', *, *, #6815, .T. ) ;
#3618=( BOUNDED_SURFACE ( )  B_SPLINE_SURFACE ( 3, 2, ( 
 ( #12873, #10400, #6848 ),
 ( #8087, #9, #919 ),
 ( #5872, #12790, #3314 ),
 ( #10553, #15095, #4390 ) ),
 .UNSPECIFIED., .F., .F., .T. ) 
 B_SPLINE_SURFACE_WITH_KNOTS ( ( 4, 4 ),
 ( 3, 3 ),
 ( -3.469446951953614189E-18, 0.006683255761480933789 ),
 ( 0.000000000000000000, 1.000000000000000000 ),
 .UNSPECIFIED. ) 
 GEOMETRIC_REPRESENTATION_ITEM ( )  RATIONAL_B_SPLINE_SURFACE ( (
 ( 1.000000000000000000, 0.6947298545087535748, 1.000000000000000000),
 ( 1.000000000000000000, 0.6996284196041377967, 1.000000000000000000),
 ( 1.000000000000000000, 0.7035788727800780240, 1.000000000000000000),
 ( 1.000000000000000000, 0.7071067811865506814, 1.000000000000000000) ) ) 
 REPRESENTATION_ITEM ( '' )  SURFACE ( )  );
#3633=ORIENTED_EDGE ( 'NONE', *, *, #5428, .T. ) ;
#3640=CARTESIAN_POINT ( 'NONE',  ( 32.45002191802005598, -59.39772283578241030, -2.758706911752222712 ) ) ;
#3644=CARTESIAN_POINT ( 'NONE',  ( 12.03298173962126150, -53.28399145779480506, -4.141535524925039624 ) ) ;
#3646=CARTESIAN_POINT ( 'NONE',  ( 29.98342429842328727, -52.28415370497024384, -3.028416065278772162 ) ) ;
#3663=CARTESIAN_POINT ( 'NONE',  ( 32.82016334605118857, -55.58238924893117172, 2.909054338253645344 ) ) ;
#3668=ORIENTED_EDGE ( 'NONE', *, *, #7814, .T. ) ;
#3673=CARTESIAN_POINT ( 'NONE',  ( 9.845387176152206266, -54.14081474687885276, 3.331943113775061693 ) ) ;
#3678=EDGE_LOOP ( 'NONE', ( #4914, #10504, #4931, #4425, #7013 ) ) ;
#3695=CARTESIAN_POINT ( 'NONE',  ( 32.64893527110322680, -58.48797006926987763, 2.754379914540435959 ) ) ;
#3696=DIRECTION ( 'NONE',  ( 0.000000000000000000, 0.000000000000000000, 1.000000000000000000 ) ) ;
#3702=CARTESIAN_POINT ( 'NONE',  ( 20.86173033120691045, -52.24929059928630437, 0.000000000000000000 ) ) ;
#3704=CARTESIAN_POINT ( 'NONE',  ( 23.36173033120691400, -85.24929059928631148, 6.000000000000001776 ) ) ;
#3712=CARTESIAN_POINT ( 'NONE',  ( 32.68132553305306232, -53.82357430177057012, 2.243931992452714130 ) ) ;
#3713=CARTESIAN_POINT ( 'NONE',  ( 33.12442251017086647, -54.47420853489484216, -2.874994438546187858 ) ) ;
#3720=VERTEX_POINT ( 'NONE', #1973 ) ;
#3731=CARTESIAN_POINT ( 'NONE',  ( 30.88245120255916021, -52.50793004641701600, 3.755530264039013577 ) ) ;
#3741=CARTESIAN_POINT ( 'NONE',  ( 8.599030766203958009, -59.21224831720011395, 1.832439066039629916 ) ) ;
#3744=AXIS2_PLACEMENT_3D ( 'NONE', #11819, #1278, #9687 ) ;
#3745=DIRECTION ( 'NONE',  ( 0.000000000000000000, 0.000000000000000000, 1.000000000000000000 ) ) ;
#3747=CIRCLE ( 'NONE', #11857, 7.000000000000000000 ) ;
#3757=CARTESIAN_POINT ( 'NONE',  ( 30.26140529969011439, -61.79747627231876095, 3.500139319474480981 ) ) ;
#3767=CYLINDRICAL_SURFACE ( 'NONE', #7181, 2.000000000000000000 ) ;
#3783=CARTESIAN_POINT ( 'NONE',  ( 8.599030766203956233, -59.21224831720010684, 1.832439066040435494 ) ) ;
#3789=LINE ( 'NONE', #6188, #921 ) ;
#3792=CARTESIAN_POINT ( 'NONE',  ( 33.62180193043921861, -56.19320768388897847, 1.864142715824113283 ) ) ;
#3793=CARTESIAN_POINT ( 'NONE',  ( 32.55528451253351108, -53.68423722363602479, -2.283982087544076389 ) ) ;
#3804=CARTESIAN_POINT ( 'NONE',  ( 29.70251902843242675, -52.24929059928631148, 4.175384597093458439 ) ) ;
#3807=VERTEX_POINT ( 'NONE', #10603 ) ;
#3812=DIRECTION ( 'NONE',  ( 0.3738365665314423159, 0.000000000000000000, -0.9274945937977119303 ) ) ;
#3814=ADVANCED_FACE ( 'NONE', ( #10532 ), #13063, .T. ) ;
#3815=FACE_OUTER_BOUND ( 'NONE', #1113, .T. ) ;
#3818=CARTESIAN_POINT ( 'NONE',  ( 8.471259741652538366, -54.75705460292326165, 2.044066819204477525 ) ) ;
#3820=CARTESIAN_POINT ( 'NONE',  ( -12.09280073291247781, -82.24929059928629727, 11.78977872328357357 ) ) ;
#3821=EDGE_LOOP ( 'NONE', ( #4973, #325, #13448, #12989 ) ) ;
#3827=CARTESIAN_POINT ( 'NONE',  ( 29.96883933646702758, -63.18892729117397522, 3.546101824483956388 ) ) ;
#3834=CARTESIAN_POINT ( 'NONE',  ( 28.59185145675412443, -64.18054652438912910, -4.118450070759198667 ) ) ;
#3836=VERTEX_POINT ( 'NONE', #6209 ) ;
#3856=CARTESIAN_POINT ( 'NONE',  ( 32.72879314807957485, -60.25563941105167487, 1.887923216546060212 ) ) ;
#3859=CARTESIAN_POINT ( 'NONE',  ( 29.35555050496136431, -52.24929059928631148, 3.199931146564417350 ) ) ;
#3860=CARTESIAN_POINT ( 'NONE',  ( 33.03498543261559206, -54.32282595323827934, -2.125007313488010308 ) ) ;
#3864=DIRECTION ( 'NONE',  ( 0.000000000000000000, 1.000000000000000000, 0.000000000000000000 ) ) ;
#3867=CARTESIAN_POINT ( 'NONE',  ( 33.38971410812750662, -58.06117559053650723, -1.821720188305476773 ) ) ;
#3868=AXIS2_PLACEMENT_3D ( 'NONE', #6890, #4265, #11580 ) ;
#3880=CARTESIAN_POINT ( 'NONE',  ( 8.948129010634172431, -57.91122518709823908, -2.751677560524413035 ) ) ;
#3886=CARTESIAN_POINT ( 'NONE',  ( 24.10826840236109803, -69.39711819508849544, -6.201611931792124111 ) ) ;
#3891=CARTESIAN_POINT ( 'NONE',  ( 20.86173033120691045, -72.24929059928631148, 0.000000000000000000 ) ) ;
#3896=EDGE_CURVE ( 'NONE', #3836, #10222, #6872, .T. ) ;
#3897=ADVANCED_FACE ( 'NONE', ( #4091 ), #13642, .F. ) ;
#3905=CARTESIAN_POINT ( 'NONE',  ( 29.10765984106813420, -64.50532980541188977, 3.862852061917652513 ) ) ;
#3910=CARTESIAN_POINT ( 'NONE',  ( 29.24098086411812147, -64.27177309650900838, -3.135762038892989878 ) ) ;
#3919=ORIENTED_EDGE ( 'NONE', *, *, #5704, .T. ) ;
#3931=CARTESIAN_POINT ( 'NONE',  ( 13.24997490312535753, -58.78531205390407877, 4.199849437504418859 ) ) ;
#3934=CARTESIAN_POINT ( 'NONE',  ( 33.31490201906242277, -54.89597349494514589, -2.779010397565622625 ) ) ;
#3950=CARTESIAN_POINT ( 'NONE',  ( 28.02673944706192088, -65.45069003752192316, -4.122770147305073074 ) ) ;
#3957=CIRCLE ( 'NONE', #4203, 0.9999999999999980016 ) ;
#3971=LINE ( 'NONE', #1596, #7794 ) ;
#3978=LINE ( 'NONE', #1681, #6068 ) ;
#3990=ORIENTED_EDGE ( 'NONE', *, *, #4861, .F. ) ;
#3998=DIRECTION ( 'NONE',  ( -0.000000000000000000, -0.000000000000000000, -1.000000000000000000 ) ) ;
#4002=CARTESIAN_POINT ( 'NONE',  ( 7.495397352420198445, -51.17708206447213115, 2.732753929628628065 ) ) ;
#4008=CARTESIAN_POINT ( 'NONE',  ( 12.61580082134606684, -64.50532980541187555, -3.862852061920813984 ) ) ;
#4009=( BOUNDED_SURFACE ( )  B_SPLINE_SURFACE ( 3, 2, ( 
 ( #11444, #680, #1839 ),
 ( #13695, #9164, #13617 ),
 ( #5467, #10160, #2146 ),
 ( #3151, #3304, #7851 ),
 ( #12543, #4451, #911 ),
 ( #1988, #6688, #7997 ) ),
 .UNSPECIFIED., .F., .F., .F. ) 
 B_SPLINE_SURFACE_WITH_KNOTS ( ( 4, 2, 4 ),
 ( 3, 3 ),
 ( 1.084202172485504434E-19, 0.001005789800061011787, 0.002011579600122023574 ),
 ( 0.000000000000000000, 1.000000000000000000 ),
 .UNSPECIFIED. ) 
 GEOMETRIC_REPRESENTATION_ITEM ( )  RATIONAL_B_SPLINE_SURFACE ( (
 ( 1.000000000000000000, 0.8308543624379425285, 1.000000000000000000),
 ( 1.000000000000000000, 0.8317114229140971648, 1.000000000000000000),
 ( 1.000000000000000000, 0.8301458553070009128, 1.000000000000000000),
 ( 1.000000000000000000, 0.8215594255314535577, 1.000000000000000000),
 ( 1.000000000000000000, 0.8147253674585736016, 1.000000000000000000),
 ( 1.000000000000000000, 0.8053615646146359275, 1.000000000000000000) ) ) 
 REPRESENTATION_ITEM ( '' )  SURFACE ( )  );
#4011=ORIENTED_EDGE ( 'NONE', *, *, #12622, .F. ) ;
#4017=CARTESIAN_POINT ( 'NONE',  ( 20.86173033120691045, -57.24929059928630437, 0.000000000000000000 ) ) ;
#4023=CARTESIAN_POINT ( 'NONE',  ( 35.09024216261268236, -47.02718879221286841, -2.731995254387835192 ) ) ;
#4026=CYLINDRICAL_SURFACE ( 'NONE', #308, 4.276034690655509785 ) ;
#4027=VERTEX_POINT ( 'NONE', #7959 ) ;
#4050=CARTESIAN_POINT ( 'NONE',  ( 29.87892709566675009, -63.30956378474007806, -2.875213255995181960 ) ) ;
#4064=PRODUCT_CONTEXT ( 'NONE', #8716, 'mechanical' ) ;
#4066=FACE_OUTER_BOUND ( 'NONE', #7365, .T. ) ;
#4068=ORIENTED_EDGE ( 'NONE', *, *, #7117, .F. ) ;
#4072=CARTESIAN_POINT ( 'NONE',  ( 11.13001753994803344, -62.42480215138046873, -2.585081138721826211 ) ) ;
#4073=EDGE_LOOP ( 'NONE', ( #1869, #5284, #5139, #13523 ) ) ;
#4076=EDGE_CURVE ( 'NONE', #13835, #7432, #7802, .T. ) ;
#4081=CARTESIAN_POINT ( 'NONE',  ( 33.25707175992479847, -58.63671300496867644, -1.826958383926200247 ) ) ;
#4082=CARTESIAN_POINT ( 'NONE',  ( 0.000000000000000000, 0.000000000000000000, 0.000000000000000000 ) ) ;
#4090=( BOUNDED_SURFACE ( )  B_SPLINE_SURFACE ( 3, 2, ( 
 ( #2162, #11540, #998 ),
 ( #10406, #14156, #8534 ),
 ( #7225, #12069, #1373 ),
 ( #228, #8316, #9771 ) ),
 .UNSPECIFIED., .F., .F., .F. ) 
 B_SPLINE_SURFACE_WITH_KNOTS ( ( 4, 4 ),
 ( 3, 3 ),
 ( -3.469446951953614189E-18, 0.006683255761480919911 ),
 ( 0.000000000000000000, 1.000000000000000000 ),
 .UNSPECIFIED. ) 
 GEOMETRIC_REPRESENTATION_ITEM ( )  RATIONAL_B_SPLINE_SURFACE ( (
 ( 1.000000000000000000, 0.7071067811865500152, 1.000000000000000000),
 ( 1.000000000000000000, 0.7035788727800782461, 1.000000000000000000),
 ( 1.000000000000000000, 0.6996284196041381298, 1.000000000000000000),
 ( 1.000000000000000000, 0.6947298545087535748, 1.000000000000000000) ) ) 
 REPRESENTATION_ITEM ( '' )  SURFACE ( )  );
#4091=FACE_OUTER_BOUND ( 'NONE', #8052, .T. ) ;
#4093=ADVANCED_FACE ( 'NONE', ( #4260 ), #10496, .T. ) ;
#4094=CIRCLE ( 'NONE', #8047, 3.999999999999999112 ) ;
#4098=CARTESIAN_POINT ( 'NONE',  ( 28.99843454536937415, -51.89470720436212048, -4.215327499024904334 ) ) ;
#4104=ORIENTED_EDGE ( 'NONE', *, *, #7251, .T. ) ;
#4118=CARTESIAN_POINT ( 'NONE',  ( 9.657637030002515388, -61.15506547911440549, 2.039555069691858513 ) ) ;
#4121=CARTESIAN_POINT ( 'NONE',  ( 20.86173033120691045, -57.24929059928630437, 0.000000000000000000 ) ) ;
#4134=CYLINDRICAL_SURFACE ( 'NONE', #7640, 3.951771890309584645 ) ;
#4142=EDGE_CURVE ( 'NONE', #14923, #5424, #5818, .T. ) ;
#4153=CARTESIAN_POINT ( 'NONE',  ( 33.62991918736606323, -56.17545244456535158, -1.862977194132048764 ) ) ;
#4155=CARTESIAN_POINT ( 'NONE',  ( 11.84453356674737101, -63.30956378474044044, -2.875213255991756700 ) ) ;
#4157=CARTESIAN_POINT ( 'NONE',  ( 33.62061467546807592, -56.17744385466402690, 1.865378520189665545 ) ) ;
#4158=VECTOR ( 'NONE', #3016, 1000.000000000000000 ) ;
#4162=CARTESIAN_POINT ( 'NONE',  ( 27.41707935315583455, -67.70775585802556407, -4.528449950254390899 ) ) ;
#4166=EDGE_CURVE ( 'NONE', #13981, #13835, #5800, .T. ) ;
#4180=CARTESIAN_POINT ( 'NONE',  ( 13.86173033120691578, -69.39711819508849544, -3.710481764567795437 ) ) ;
#4182=CARTESIAN_POINT ( 'NONE',  ( 11.13001753994774212, -62.42480215138011346, 2.585081138721638361 ) ) ;
#4184=CARTESIAN_POINT ( 'NONE',  ( 10.43256186016586184, -53.71411213207043289, 3.559347964322298719 ) ) ;
#4185=FACE_OUTER_BOUND ( 'NONE', #7947, .T. ) ;
#4190=AXIS2_PLACEMENT_3D ( 'NONE', #10593, #7205, #8449 ) ;
#4198=EDGE_CURVE ( 'NONE', #8129, #14139, #5750, .T. ) ;
#4202=CARTESIAN_POINT ( 'NONE',  ( 27.86203511185233594, -69.48056866272028742, -4.214447830835834630 ) ) ;
#4203=AXIS2_PLACEMENT_3D ( 'NONE', #6960, #12969, #7112 ) ;
#4208=CARTESIAN_POINT ( 'NONE',  ( 11.41872426162122345, -52.33170319195679099, -3.962365649671490075 ) ) ;
#4215=AXIS2_PLACEMENT_3D ( 'NONE', #14941, #13785, #11171 ) ;
#4229=CARTESIAN_POINT ( 'NONE',  ( 16.53849081582479386, -69.39711819508849544, 5.637959728397555992 ) ) ;
#4230=CARTESIAN_POINT ( 'NONE',  ( 12.48247979829434584, -64.27177309650687675, -3.135762038895900439 ) ) ;
#4233=EDGE_LOOP ( 'NONE', ( #4788, #12929, #10018, #8945 ) ) ;
#4238=CARTESIAN_POINT ( 'NONE',  ( 28.09009917991004812, -65.27414832489905905, -4.302972696997105828 ) ) ;
#4241=DIRECTION ( 'NONE',  ( 0.000000000000000000, 1.000000000000000000, 0.000000000000000000 ) ) ;
#4247=CARTESIAN_POINT ( 'NONE',  ( 29.69047892279256118, -53.28399145779480506, 4.141535524925028966 ) ) ;
#4252=CARTESIAN_POINT ( 'NONE',  ( 31.88156390563087683, -61.30062302791112927, 2.840369378987805060 ) ) ;
#4253=EDGE_CURVE ( 'NONE', #3440, #15191, #1032, .T. ) ;
#4255=CARTESIAN_POINT ( 'NONE',  ( 23.10474973039556801, -52.24929059928630437, -5.564967562786270250 ) ) ;
#4256=DIRECTION ( 'NONE',  ( 0.9744556954135528137, 0.2245798247307385087, -0.000000000000000000 ) ) ;
#4260=FACE_OUTER_BOUND ( 'NONE', #9077, .T. ) ;
#4261=CARTESIAN_POINT ( 'NONE',  ( 10.27153280171312666, -52.79510901551753221, 2.616251790959217782 ) ) ;
#4262=DIRECTION ( 'NONE',  ( 0.000000000000000000, 0.000000000000000000, 1.000000000000000000 ) ) ;
#4265=DIRECTION ( 'NONE',  ( -0.9421718071228325497, -3.620235254251614364E-16, -0.3351302520855077294 ) ) ;
#4266=ORIENTED_EDGE ( 'NONE', *, *, #13085, .F. ) ;
#4267=CARTESIAN_POINT ( 'NONE',  ( 8.597635011448852893, -59.20619211347771227, 2.502190571104538463 ) ) ;
#4271=CARTESIAN_POINT ( 'NONE',  ( 31.88917822179636374, -54.14192065903539230, -3.328125142887244703 ) ) ;
#4276=CARTESIAN_POINT ( 'NONE',  ( 53.81626139532630759, -85.24929059928631148, 11.78977872328355048 ) ) ;
#4281=CARTESIAN_POINT ( 'NONE',  ( 8.090330977888115171, -56.40460476644708621, -2.550424528238877553 ) ) ;
#4282=DIRECTION ( 'NONE',  ( -0.7546336727145983581, 0.5961293309129265250, 0.2741493039031521195 ) ) ;
#4289=ORIENTED_EDGE ( 'NONE', *, *, #881, .F. ) ;
#4300=CARTESIAN_POINT ( 'NONE',  ( 33.63314816004646701, -56.83321641073668218, -1.823854045754459641 ) ) ;
#4302=CARTESIAN_POINT ( 'NONE',  ( 13.41074896738031264, -66.37912134691028143, -3.509717431437874069 ) ) ;
#4305=B_SPLINE_CURVE_WITH_KNOTS ( 'NONE', 3,
 ( #624, #5329, #13339, #13268 ),
 .UNSPECIFIED., .F., .F.,
 ( 4, 4 ),
 ( 0.000000000000000000, 0.001771361151111836745 ),
 .UNSPECIFIED. ) ;
#4319=CARTESIAN_POINT ( 'NONE',  ( 12.06345512429583344, -63.57773214734891098, 2.964070158660694787 ) ) ;
#4333=EDGE_CURVE ( 'NONE', #11968, #625, #11380, .T. ) ;
#4337=CARTESIAN_POINT ( 'NONE',  ( 9.664560468771329127, -61.13673569060787827, -2.043233430234987935 ) ) ;
#4348=CARTESIAN_POINT ( 'NONE',  ( 17.36157654472071599, -73.69234276600508338, -6.062089035220971311 ) ) ;
#4349=ORIENTED_EDGE ( 'NONE', *, *, #1349, .F. ) ;
#4352=CARTESIAN_POINT ( 'NONE',  ( 12.91422301979531717, -63.78832907041026345, -4.037694147267451683 ) ) ;
#4353=FACE_OUTER_BOUND ( 'NONE', #9221, .T. ) ;
#4358=LINE ( 'NONE', #12523, #8690 ) ;
#4366=CARTESIAN_POINT ( 'NONE',  ( 8.129701836179927810, -57.17378631614188578, -2.501045389182539935 ) ) ;
#4369=ORIENTED_EDGE ( 'NONE', *, *, #3054, .F. ) ;
#4387=CARTESIAN_POINT ( 'NONE',  ( 8.821484763567294607, -57.33450387999030795, 2.749014434309869248 ) ) ;
#4390=CARTESIAN_POINT ( 'NONE',  ( 23.47858629692699139, -53.24929059928630437, 6.492462156583989952 ) ) ;
#4391=CARTESIAN_POINT ( 'NONE',  ( 32.59721271199144610, -59.08477032946249352, 2.725562014970989377 ) ) ;
#4392=VERTEX_POINT ( 'NONE', #7933 ) ;
#4393=CARTESIAN_POINT ( 'NONE',  ( 33.52366768382368889, -57.47994873761393819, 2.501453769636589275 ) ) ;
#4395=ORIENTED_EDGE ( 'NONE', *, *, #882, .T. ) ;
#4398=FACE_OUTER_BOUND ( 'NONE', #11661, .T. ) ;
#4403=DIRECTION ( 'NONE',  ( 0.000000000000000000, -1.000000000000000000, 0.000000000000000000 ) ) ;
#4408=CARTESIAN_POINT ( 'NONE',  ( 33.12582565096496268, -59.20619211347771937, 2.502190571104481176 ) ) ;
#4417=CARTESIAN_POINT ( 'NONE',  ( 8.994667514334258485, -60.25563941105167487, -1.887923216546042449 ) ) ;
#4418=DIRECTION ( 'NONE',  ( -0.000000000000000000, 1.000000000000000000, -0.000000000000000000 ) ) ;
#4425=ORIENTED_EDGE ( 'NONE', *, *, #1180, .F. ) ;
#4435=DIRECTION ( 'NONE',  ( -0.000000000000000000, -0.000000000000000000, -1.000000000000000000 ) ) ;
#4436=CARTESIAN_POINT ( 'NONE',  ( 27.33509234239454244, -69.49659648540917090, -4.497058153269716918 ) ) ;
#4437=ORIENTED_EDGE ( 'NONE', *, *, #9364, .T. ) ;
#4439=CARTESIAN_POINT ( 'NONE',  ( 10.55748904889333772, -52.62785358159961646, -3.652922677138590757 ) ) ;
#4451=CARTESIAN_POINT ( 'NONE',  ( 9.539473796687049756, -61.03341231845509895, -2.731818205567035474 ) ) ;
#4455=VECTOR ( 'NONE', #11492, 1000.000000000000000 ) ;
#4466=AXIS2_PLACEMENT_3D ( 'NONE', #7434, #12127, #572 ) ;
#4480=CARTESIAN_POINT ( 'NONE',  ( 32.52281604437752804, -59.06479067038041109, -2.757123406423310552 ) ) ;
#4484=CARTESIAN_POINT ( 'NONE',  ( 30.63989068920077230, -53.42334933900650640, 3.800563870772192043 ) ) ;
#4489=ADVANCED_FACE ( 'NONE', ( #88 ), #3767, .T. ) ;
#4490=CARTESIAN_POINT ( 'NONE',  ( 32.36444917618072736, -60.82759157437160979, 1.965556376685483331 ) ) ;
#4494=DIRECTION ( 'NONE',  ( -0.2245798247307385087, 0.9744556954135528137, 0.000000000000000000 ) ) ;
#4496=EDGE_LOOP ( 'NONE', ( #8466, #11675, #11635, #10550 ) ) ;
#4504=CIRCLE ( 'NONE', #13120, 0.9999999999999991118 ) ;
#4506=DIRECTION ( 'NONE',  ( 0.000000000000000000, 1.000000000000000000, 0.000000000000000000 ) ) ;
#4508=EDGE_LOOP ( 'NONE', ( #7540, #6040, #6962, #8539 ) ) ;
#4509=CARTESIAN_POINT ( 'NONE',  ( 13.69731538040242746, -65.45139068073372357, -4.123085412756658741 ) ) ;
#4513=CARTESIAN_POINT ( 'NONE',  ( 11.45350991191545553, -61.78874994510978524, -3.497001979624778212 ) ) ;
#4514=B_SPLINE_CURVE_WITH_KNOTS ( 'NONE', 3,
 ( #7355, #12044, #10904, #7433 ),
 .UNSPECIFIED., .F., .F.,
 ( 4, 4 ),
 ( 0.0005996816226312184136, 0.004245596575621797542 ),
 .UNSPECIFIED. ) ;
#4516=CYLINDRICAL_SURFACE ( 'NONE', #8527, 2.000000000000000000 ) ;
#4524=CARTESIAN_POINT ( 'NONE',  ( 9.275519748983422019, -53.56780286158462445, -2.317958153236276964 ) ) ;
#4529=ORIENTED_EDGE ( 'NONE', *, *, #6621, .T. ) ;
#4541=DIRECTION ( 'NONE',  ( 0.000000000000000000, 0.000000000000000000, 1.000000000000000000 ) ) ;
#4543=CARTESIAN_POINT ( 'NONE',  ( 33.58940973320519419, -55.84353942689658368, -1.893207994803262739 ) ) ;
#4546=CARTESIAN_POINT ( 'NONE',  ( 28.15716758062500702, -63.36896821088274123, 4.156457392287215669 ) ) ;
#4561=CARTESIAN_POINT ( 'NONE',  ( 32.37590170700519110, -54.69585338401581964, 3.125080077088496555 ) ) ;
#4568=CARTESIAN_POINT ( 'NONE',  ( 32.10922531551839398, -61.48375833294921478, -2.718831331512520322 ) ) ;
#4575=CARTESIAN_POINT ( 'NONE',  ( 13.77965687262195260, -67.87804980504323282, 4.252496648654521039 ) ) ;
#4582=CARTESIAN_POINT ( 'NONE',  ( 13.86173033120691223, -69.39711819508849544, 2.500000000000000000 ) ) ;
#4584=CARTESIAN_POINT ( 'NONE',  ( 6.988058422621596932, -48.72530132304424910, -2.733088102048180978 ) ) ;
#4590=( NAMED_UNIT ( * ) SI_UNIT ( $, .STERADIAN. ) SOLID_ANGLE_UNIT ( ) );
#4591=CARTESIAN_POINT ( 'NONE',  ( 18.08359295236611786, -58.63441909321038281, -6.426091441073433330 ) ) ;
#4599=CARTESIAN_POINT ( 'NONE',  ( 8.097303543835579376, -56.24990207478561643, -2.565511669097837455 ) ) ;
#4608=CIRCLE ( 'NONE', #13217, 0.9999999999999996669 ) ;
#4613=CIRCLE ( 'NONE', #12475, 7.000000000000000000 ) ;
#4625=CARTESIAN_POINT ( 'NONE',  ( 23.59140218558529867, -57.03285117761353717, 6.445925775545360281 ) ) ;
#4628=CARTESIAN_POINT ( 'NONE',  ( 12.36791015745245836, -52.24929059928631148, 3.199931146564429341 ) ) ;
#4635=CARTESIAN_POINT ( 'NONE',  ( 8.201103799357259305, -57.48563641131178770, 1.816685854991402893 ) ) ;
#4640=CARTESIAN_POINT ( 'NONE',  ( 8.873138538923161178, -60.06401564186453612, 1.862089353234911204 ) ) ;
#4642=CARTESIAN_POINT ( 'NONE',  ( 12.36791015745245836, -52.24929059928631148, -3.199931146564426232 ) ) ;
#4650=ORIENTED_EDGE ( 'NONE', *, *, #11318, .F. ) ;
#4658=LINE ( 'NONE', #1107, #10516 ) ;
#4662=CARTESIAN_POINT ( 'NONE',  ( 32.39494368350905518, -53.50439862579374761, 3.186601206341092674 ) ) ;
#4664=CARTESIAN_POINT ( 'NONE',  ( 13.56629308258002098, -63.36896821090397225, -4.156457390613502945 ) ) ;
#4669=ORIENTED_EDGE ( 'NONE', *, *, #580, .F. ) ;
#4678=CARTESIAN_POINT ( 'NONE',  ( 8.201103799357259305, -57.48563641131178770, -1.816685854991388682 ) ) ;
#4680=FACE_OUTER_BOUND ( 'NONE', #3515, .T. ) ;
#4691=CARTESIAN_POINT ( 'NONE',  ( 20.86173033120691045, -96.56299909827106376, 0.000000000000000000 ) ) ;
#4696=( BOUNDED_SURFACE ( )  B_SPLINE_SURFACE ( 3, 2, ( 
 ( #4255, #3337, #13572 ),
 ( #5575, #13728, #3103 ),
 ( #1944, #12416, #10344 ),
 ( #3041, #12652, #12347 ) ),
 .UNSPECIFIED., .F., .F., .F. ) 
 B_SPLINE_SURFACE_WITH_KNOTS ( ( 4, 4 ),
 ( 3, 3 ),
 ( 3.469446951953614189E-18, 0.006683255761480919911 ),
 ( 0.000000000000000000, 1.000000000000000000 ),
 .UNSPECIFIED. ) 
 GEOMETRIC_REPRESENTATION_ITEM ( )  RATIONAL_B_SPLINE_SURFACE ( (
 ( 1.000000000000000000, 0.7071067811865500152, 1.000000000000000000),
 ( 1.000000000000000000, 0.7035788727800790232, 1.000000000000000000),
 ( 1.000000000000000000, 0.6996284196041374637, 1.000000000000000000),
 ( 1.000000000000000000, 0.6947298545087537969, 1.000000000000000000) ) ) 
 REPRESENTATION_ITEM ( '' )  SURFACE ( )  );
#4698=DIRECTION ( 'NONE',  ( 0.000000000000000000, 0.000000000000000000, 1.000000000000000000 ) ) ;
#4700=ADVANCED_FACE ( 'NONE', ( #4398 ), #6706, .F. ) ;
#4710=B_SPLINE_CURVE_WITH_KNOTS ( 'NONE', 3,
 ( #188, #1188, #11800, #1258, #3499, #8201 ),
 .UNSPECIFIED., .F., .F.,
 ( 4, 2, 4 ),
 ( 0.001000432843099107339, 0.009082381923694659437, 0.01716433100429023278 ),
 .UNSPECIFIED. ) ;
#4737=CARTESIAN_POINT ( 'NONE',  ( 14.31939787082484727, -67.79239290436629517, 4.531617596076316090 ) ) ;
#4742=DIRECTION ( 'NONE',  ( 0.000000000000000000, -1.000000000000000000, 0.000000000000000000 ) ) ;
#4744=EDGE_CURVE ( 'NONE', #2756, #5424, #3747, .T. ) ;
#4745=CARTESIAN_POINT ( 'NONE',  ( 30.62910135305399351, -53.42013688713479524, 3.804487959019970056 ) ) ;
#4747=CARTESIAN_POINT ( 'NONE',  ( 13.86173033120691223, -69.39711819508849544, 2.500000000000000000 ) ) ;
#4750=ORIENTED_EDGE ( 'NONE', *, *, #13281, .F. ) ;
#4752=ORIENTED_EDGE ( 'NONE', *, *, #5951, .T. ) ;
#4753=VERTEX_POINT ( 'NONE', #12486 ) ;
#4756=DIRECTION ( 'NONE',  ( 0.000000000000000000, -1.000000000000000000, 0.000000000000000000 ) ) ;
#4757=AXIS2_PLACEMENT_3D ( 'NONE', #12137, #11048, #1592 ) ;
#4765=VERTEX_POINT ( 'NONE', #3171 ) ;
#4769=CARTESIAN_POINT ( 'NONE',  ( 10.23047706855496308, -60.71197230342421136, -3.050751728647428607 ) ) ;
#4770=ORIENTED_EDGE ( 'NONE', *, *, #5411, .F. ) ;
#4772=AXIS2_PLACEMENT_3D ( 'NONE', #1967, #13522, #2989 ) ;
#4776=CARTESIAN_POINT ( 'NONE',  ( 25.17145219045130489, -52.24929059928630437, -4.731961142181946300 ) ) ;
#4788=ORIENTED_EDGE ( 'NONE', *, *, #14249, .F. ) ;
#4790=CARTESIAN_POINT ( 'NONE',  ( 8.597635011448856446, -59.20619211347771937, 2.502190571104474959 ) ) ;
#4797=CARTESIAN_POINT ( 'NONE',  ( 32.86846178545243902, -54.08202937160073986, 2.181355823101601477 ) ) ;
#4798=CARTESIAN_POINT ( 'NONE',  ( 32.50723669307611630, -54.89772082965748012, -3.066133849897850983 ) ) ;
#4803=DIRECTION ( 'NONE',  ( -0.000000000000000000, -0.000000000000000000, -1.000000000000000000 ) ) ;
#4812=AXIS2_PLACEMENT_3D ( 'NONE', #8624, #1558, #12167 ) ;
#4814=VECTOR ( 'NONE', #15183, 1000.000000000000000 ) ;
#4815=CARTESIAN_POINT ( 'NONE',  ( 32.09796538084800943, -53.24070755262462740, 2.425727701578423989 ) ) ;
#4820=CARTESIAN_POINT ( 'NONE',  ( 8.599030766203958009, -59.21224831720011395, 1.832439066039629916 ) ) ;
#4821=EDGE_CURVE ( 'NONE', #5130, #304, #6902, .T. ) ;
#4826=CARTESIAN_POINT ( 'NONE',  ( 13.86173033120691223, -68.61243380581731799, -3.657093847832751710 ) ) ;
#4836=ORIENTED_EDGE ( 'NONE', *, *, #14223, .F. ) ;
#4837=CARTESIAN_POINT ( 'NONE',  ( 28.33202942550559555, -66.31583591551219570, 4.137138225905043321 ) ) ;
#4839=ORIENTED_EDGE ( 'NONE', *, *, #8668, .F. ) ;
#4845=AXIS2_PLACEMENT_3D ( 'NONE', #4017, #9882, #7722 ) ;
#4849=ORIENTED_EDGE ( 'NONE', *, *, #4, .F. ) ;
#4855=CARTESIAN_POINT ( 'NONE',  ( -12.09280073291247781, 0.000000000000000000, 11.78977872328357357 ) ) ;
#4861=EDGE_CURVE ( 'NONE', #11986, #3440, #9116, .T. ) ;
#4865=CARTESIAN_POINT ( 'NONE',  ( 27.95143033160315937, -67.83931925369923022, 3.638954064322518889 ) ) ;
#4871=AXIS2_PLACEMENT_3D ( 'NONE', #10126, #14812, #4262 ) ;
#4875=CARTESIAN_POINT ( 'NONE',  ( 32.11820540151424552, -53.25766581158782742, 2.419604383416593674 ) ) ;
#4883=VECTOR ( 'NONE', #11807, 1000.000000000000000 ) ;
#4892=CARTESIAN_POINT ( 'NONE',  ( 33.57093241131959616, -55.78447712832138450, 2.622266312280598033 ) ) ;
#4896=VERTEX_POINT ( 'NONE', #10793 ) ;
#4905=CARTESIAN_POINT ( 'NONE',  ( 8.126138517945966200, -57.16036077483330047, 1.814506011345170755 ) ) ;
#4912=ORIENTED_EDGE ( 'NONE', *, *, #5007, .F. ) ;
#4914=ORIENTED_EDGE ( 'NONE', *, *, #7117, .T. ) ;
#4915=ADVANCED_FACE ( 'NONE', ( #4066 ), #9941, .F. ) ;
#4928=CARTESIAN_POINT ( 'NONE',  ( 18.03113812440135888, 0.000000000000000000, 4.472107801411127959 ) ) ;
#4931=ORIENTED_EDGE ( 'NONE', *, *, #9975, .F. ) ;
#4940=DIRECTION ( 'NONE',  ( 0.000000000000000000, -0.000000000000000000, -1.000000000000000000 ) ) ;
#4941=CARTESIAN_POINT ( 'NONE',  ( 31.13618595441765180, -61.88944072237682548, 2.366779157396534661 ) ) ;
#4942=CARTESIAN_POINT ( 'NONE',  ( 21.74884261173415467, -82.24929059928629727, -6.000000000000000888 ) ) ;
#4947=CARTESIAN_POINT ( 'NONE',  ( 30.59878209274603478, -52.42197922347948946, 2.858153496903512725 ) ) ;
#4948=CARTESIAN_POINT ( 'NONE',  ( 29.70251902843241965, -52.24929059928630437, -4.175384597093456662 ) ) ;
#4964=VECTOR ( 'NONE', #8207, 1000.000000000000000 ) ;
#4968=CARTESIAN_POINT ( 'NONE',  ( 31.45480550940234821, -52.78690463904968055, 2.615816816689916724 ) ) ;
#4973=ORIENTED_EDGE ( 'NONE', *, *, #9436, .F. ) ;
#4979=DIRECTION ( 'NONE',  ( 0.000000000000000000, 0.000000000000000000, -1.000000000000000000 ) ) ;
#4985=CARTESIAN_POINT ( 'NONE',  ( 23.36173033120691400, -82.24929059928629727, -6.000000000000000888 ) ) ;
#4993=CARTESIAN_POINT ( 'NONE',  ( 9.412906046440658869, -59.69871785856275892, -2.790504257380244546 ) ) ;
#5004=CARTESIAN_POINT ( 'NONE',  ( 29.24282639220472291, -63.10178406536538631, -3.876738539648747928 ) ) ;
#5007=EDGE_CURVE ( 'NONE', #5832, #9444, #5310, .T. ) ;
#5024=CARTESIAN_POINT ( 'NONE',  ( 17.36157654472070888, -73.69234276600499811, 6.062089035220985522 ) ) ;
#5026=CARTESIAN_POINT ( 'NONE',  ( 33.12442989620986822, -59.21224831720011395, 1.832439066039631914 ) ) ;
#5030=CARTESIAN_POINT ( 'NONE',  ( 32.69777265694848722, -53.84505747417108523, -3.062469901903030589 ) ) ;
#5041=CARTESIAN_POINT ( 'NONE',  ( 27.33382790127957662, -69.39711819508849544, -4.502057496415715399 ) ) ;
#5058=CARTESIAN_POINT ( 'NONE',  ( 8.782543352270323567, -56.07132046089833466, 2.830553478268754031 ) ) ;
#5067=CARTESIAN_POINT ( 'NONE',  ( 28.79421079956515683, -63.81378734511702788, 4.043274055230560826 ) ) ;
#5071=CARTESIAN_POINT ( 'NONE',  ( 20.86173033120691045, -57.24929059928630437, -3.000000000000000888 ) ) ;
#5073=CARTESIAN_POINT ( 'NONE',  ( 30.26140529968839843, -61.79747627231853357, -3.500139319475241262 ) ) ;
#5095=CARTESIAN_POINT ( 'NONE',  ( 12.57704357998833089, -50.05591495609738217, 4.211963358982736771 ) ) ;
#5100=CARTESIAN_POINT ( 'NONE',  ( 32.23959774372725207, -53.36427686165168893, 2.382617577203031800 ) ) ;
#5105=ORIENTED_EDGE ( 'NONE', *, *, #9436, .T. ) ;
#5107=PLANE ( 'NONE',  #1463 ) ;
#5108=CIRCLE ( 'NONE', #10514, 31.00000000000000000 ) ;
#5117=VECTOR ( 'NONE', #6785, 1000.000000000000000 ) ;
#5119=CARTESIAN_POINT ( 'NONE',  ( 34.22806330994987434, -51.17708206442508612, -2.732753929480980837 ) ) ;
#5130=VERTEX_POINT ( 'NONE', #12544 ) ;
#5135=CARTESIAN_POINT ( 'NONE',  ( -12.09280073291247426, -82.24929059928629727, -11.78977872328358067 ) ) ;
#5139=ORIENTED_EDGE ( 'NONE', *, *, #9322, .F. ) ;
#5140=CARTESIAN_POINT ( 'NONE',  ( 28.60124718008176359, -65.57050171853848042, 4.044987206835600091 ) ) ;
#5145=CARTESIAN_POINT ( 'NONE',  ( 27.94158133900257113, -67.90279320104600913, -3.641642753169207936 ) ) ;
#5154=ADVANCED_FACE ( 'NONE', ( #12390, #834 ), #3226, .F. ) ;
#5170=CARTESIAN_POINT ( 'NONE',  ( 13.65275068252246449, -65.32322779889733511, -4.310009693574635925 ) ) ;
#5176=B_SPLINE_CURVE_WITH_KNOTS ( 'NONE', 3,
 ( #9066, #1976, #6750, #9155 ),
 .UNSPECIFIED., .F., .F.,
 ( 4, 4 ),
 ( 0.000000000000000000, 0.001771943201165730340 ),
 .UNSPECIFIED. ) ;
#5183=CARTESIAN_POINT ( 'NONE',  ( 27.81150698810987265, -69.39711819508849544, -3.980554831151301265 ) ) ;
#5184=( BOUNDED_SURFACE ( )  B_SPLINE_SURFACE ( 3, 2, ( 
 ( #9335, #14026, #8187 ),
 ( #8341, #3561, #8266 ),
 ( #9493, #12956, #12890 ),
 ( #2407, #1247, #5958 ),
 ( #3640, #7022, #11868 ),
 ( #4480, #9187, #13952 ) ),
 .UNSPECIFIED., .F., .F., .F. ) 
 B_SPLINE_SURFACE_WITH_KNOTS ( ( 4, 2, 4 ),
 ( 3, 3 ),
 ( -6.505213034913026604E-18, 0.001008510999900119739, 0.002017021999800245984 ),
 ( 0.000000000000000000, 1.000000000000000000 ),
 .UNSPECIFIED. ) 
 GEOMETRIC_REPRESENTATION_ITEM ( )  RATIONAL_B_SPLINE_SURFACE ( (
 ( 1.000000000000000000, 0.8053615646146046192, 1.000000000000000000),
 ( 1.000000000000000000, 0.8146689552414230207, 1.000000000000000000),
 ( 1.000000000000000000, 0.8215765256475128231, 1.000000000000000000),
 ( 1.000000000000000000, 0.8301698670438529826, 1.000000000000000000),
 ( 1.000000000000000000, 0.8316880482410894393, 1.000000000000000000),
 ( 1.000000000000000000, 0.8308543624379411963, 1.000000000000000000) ) ) 
 REPRESENTATION_ITEM ( '' )  SURFACE ( )  );
#5186=CARTESIAN_POINT ( 'NONE',  ( 29.24198010098109890, -64.22824823034754615, -3.135769320951036221 ) ) ;
#5205=DIRECTION ( 'NONE',  ( -0.9744556954135545901, -0.2245798247307308204, 0.000000000000000000 ) ) ;
#5208=ORIENTED_EDGE ( 'NONE', *, *, #13504, .F. ) ;
#5211=CARTESIAN_POINT ( 'NONE',  ( 29.69047892279255407, -53.28399145779480506, -4.141535524925019196 ) ) ;
#5212=ORIENTED_EDGE ( 'NONE', *, *, #11700, .T. ) ;
#5215=EDGE_LOOP ( 'NONE', ( #12306, #13549, #10979, #7371 ) ) ;
#5222=CARTESIAN_POINT ( 'NONE',  ( 30.84433510184662097, -61.22098757969241944, -3.286659897588250612 ) ) ;
#5223=ORIENTED_EDGE ( 'NONE', *, *, #14223, .T. ) ;
#5226=AXIS2_PLACEMENT_3D ( 'NONE', #12781, #10465, #14005 ) ;
#5250=CARTESIAN_POINT ( 'NONE',  ( 12.36791015745245836, -52.24929059928631148, 3.199931146564429341 ) ) ;
#5254=B_SPLINE_CURVE_WITH_KNOTS ( 'NONE', 3,
 ( #11260, #4180, #3045, #13418, #2882, #7580, #716, #5423 ),
 .UNSPECIFIED., .F., .F.,
 ( 4, 2, 2, 4 ),
 ( 0.000000000000000000, 0.0002685324218445791621, 0.0005370648436891570232, 0.001074129687378310794 ),
 .UNSPECIFIED. ) ;
#5259=CARTESIAN_POINT ( 'NONE',  ( 29.35555050496136431, -52.24929059928631148, -3.199931146564432449 ) ) ;
#5264=EDGE_CURVE ( 'NONE', #10195, #12779, #6450, .T. ) ;
#5269=CARTESIAN_POINT ( 'NONE',  ( 28.25575485889338978, -61.89598878741227139, -4.173736770051541534 ) ) ;
#5275=ORIENTED_EDGE ( 'NONE', *, *, #10456, .T. ) ;
#5277=ADVANCED_FACE ( 'NONE', ( #2309 ), #1892, .T. ) ;
#5280=CARTESIAN_POINT ( 'NONE',  ( 12.36791015745246547, -52.24929059928630437, 3.199931146564424456 ) ) ;
#5284=ORIENTED_EDGE ( 'NONE', *, *, #1968, .F. ) ;
#5286=CARTESIAN_POINT ( 'NONE',  ( 20.86173033120691045, -53.24929059928630437, 0.000000000000000000 ) ) ;
#5287=ORIENTED_EDGE ( 'NONE', *, *, #9975, .T. ) ;
#5296=CARTESIAN_POINT ( 'NONE',  ( 29.65531183511549074, -63.62021712492606440, -2.966460067271383672 ) ) ;
#5300=CARTESIAN_POINT ( 'NONE',  ( 3.703153296433914665, -69.39711819508849544, 2.500000000000000000 ) ) ;
#5308=EDGE_CURVE ( 'NONE', #13577, #12159, #2684, .T. ) ;
#5310=LINE ( 'NONE', #11017, #6686 ) ;
#5319=CARTESIAN_POINT ( 'NONE',  ( 13.00536048170743797, -65.29678988936899486, -3.348867343500126825 ) ) ;
#5322=CARTESIAN_POINT ( 'NONE',  ( 33.63308522438084935, -56.83262086368724653, 1.823905708653747348 ) ) ;
#5323=B_SPLINE_CURVE_WITH_KNOTS ( 'NONE', 3,
 ( #258, #6034, #7255, #10719, #14262, #1249, #7105, #5804, #2412, #9495, #11792, #10572, #5961, #1331 ),
 .UNSPECIFIED., .F., .F.,
 ( 4, 2, 2, 2, 2, 2, 4 ),
 ( 0.000000000000000000, 0.002515995007885566369, 0.003773992511828368635, 0.005031990015771170902, 0.006289987519713973602, 0.007547985023656774567, 0.01006398003154241119 ),
 .UNSPECIFIED. ) ;
#5329=CARTESIAN_POINT ( 'NONE',  ( 9.074525391310594102, -58.48797006926988473, -2.754379914540418639 ) ) ;
#5330=ORIENTED_EDGE ( 'NONE', *, *, #9364, .F. ) ;
#5334=CARTESIAN_POINT ( 'NONE',  ( 27.41385764376421363, -69.39711819508850965, -4.459166325353804083 ) ) ;
#5340=CARTESIAN_POINT ( 'NONE',  ( 32.59856662516318693, -59.08346394664149415, -2.725125706471997145 ) ) ;
#5350=CARTESIAN_POINT ( 'NONE',  ( 8.599030766203958009, -59.21224831720011395, -1.832439066039622144 ) ) ;
#5351=CARTESIAN_POINT ( 'NONE',  ( 12.03298173962126860, -53.28399145779480506, 4.141535524925031631 ) ) ;
#5376=LINE ( 'NONE', #7839, #95 ) ;
#5392=ORIENTED_EDGE ( 'NONE', *, *, #264, .F. ) ;
#5397=CARTESIAN_POINT ( 'NONE',  ( 12.48063427020827021, -63.10178406536854112, -3.876738539648207471 ) ) ;
#5411=EDGE_CURVE ( 'NONE', #13900, #10942, #8538, .T. ) ;
#5416=CARTESIAN_POINT ( 'NONE',  ( 23.47466359740176145, -53.10810670090258867, -6.494041865157049287 ) ) ;
#5419=CARTESIAN_POINT ( 'NONE',  ( 11.26881178693570362, -52.38369591842261030, 2.898182089495347391 ) ) ;
#5423=CARTESIAN_POINT ( 'NONE',  ( 14.38963276113425138, -69.39711819508849544, -4.502057496415714510 ) ) ;
#5424=VERTEX_POINT ( 'NONE', #2907 ) ;
#5425=CARTESIAN_POINT ( 'NONE',  ( 10.00023835250150483, -61.42570632716525125, -2.132522520905374197 ) ) ;
#5428=EDGE_CURVE ( 'NONE', #2922, #12406, #8215, .T. ) ;
#5430=CYLINDRICAL_SURFACE ( 'NONE', #4871, 31.00000000000000000 ) ;
#5438=CARTESIAN_POINT ( 'NONE',  ( 32.51083376785603463, -54.90380519981211194, -3.064473585392911481 ) ) ;
#5446=VERTEX_POINT ( 'NONE', #7908 ) ;
#5448=CIRCLE ( 'NONE', #7421, 3.999999999999999112 ) ;
#5453=CARTESIAN_POINT ( 'NONE',  ( 9.668720703607657896, -54.31361072226496134, -3.260388240305699181 ) ) ;
#5465=CARTESIAN_POINT ( 'NONE',  ( 27.86173033120691045, -69.39711819508849544, 3.619682905202613377 ) ) ;
#5467=CARTESIAN_POINT ( 'NONE',  ( 9.400986902400736867, -59.70726391082678930, -2.784470044084383478 ) ) ;
#5469=VECTOR ( 'NONE', #13302, 1000.000000000000000 ) ;
#5479=CARTESIAN_POINT ( 'NONE',  ( 12.92924986285064115, -63.81378734511702788, -4.043274055231452557 ) ) ;
#5480=EDGE_CURVE ( 'NONE', #10942, #12159, #70, .T. ) ;
#5482=CARTESIAN_POINT ( 'NONE',  ( 33.55155325696184576, -55.68585955703496637, 1.912302604851222387 ) ) ;
#5485=EDGE_CURVE ( 'NONE', #6079, #3807, #4358, .T. ) ;
#5488=CARTESIAN_POINT ( 'NONE',  ( 27.32685193182241079, -68.54636829475870741, -4.542647641079959442 ) ) ;
#5497=CARTESIAN_POINT ( 'NONE',  ( 23.36173033120691400, -85.24929059928631148, -6.000000000000000888 ) ) ;
#5506=CARTESIAN_POINT ( 'NONE',  ( 12.36791015745245836, -52.24929059928631148, 3.199931146564429341 ) ) ;
#5513=CARTESIAN_POINT ( 'NONE',  ( 13.50577566551452513, -66.70046270226335139, 4.174231074480405645 ) ) ;
#5515=CARTESIAN_POINT ( 'NONE',  ( 33.63091130056225353, -56.19153130592571443, -1.861773613859164511 ) ) ;
#5516=CARTESIAN_POINT ( 'NONE',  ( 9.573486461617511267, -58.98766849246937483, 1.832439066040226106 ) ) ;
#5520=CARTESIAN_POINT ( 'NONE',  ( 13.88366620244440064, -68.65220048136326625, -4.053998922580050568 ) ) ;
#5521=ORIENTED_EDGE ( 'NONE', *, *, #5704, .F. ) ;
#5524=CARTESIAN_POINT ( 'NONE',  ( 27.40406279159242331, -67.79239290436652254, 4.531617596074583254 ) ) ;
#5526=ADVANCED_FACE ( 'NONE', ( #6665 ), #6744, .T. ) ;
#5530=CARTESIAN_POINT ( 'NONE',  ( 17.09549820959326638, -96.56299909827106376, -1.347403282660980084 ) ) ;
#5533=CARTESIAN_POINT ( 'NONE',  ( 10.83605996619203715, -52.52081589074905565, -2.777424068826388925 ) ) ;
#5534=CARTESIAN_POINT ( 'NONE',  ( 10.62011700622559474, -60.64100864355887666, -2.132522520905393737 ) ) ;
#5538=ORIENTED_EDGE ( 'NONE', *, *, #5007, .T. ) ;
#5544=CARTESIAN_POINT ( 'NONE',  ( 12.03298173962126150, -53.28399145779480506, -4.141535524925039624 ) ) ;
#5549=CARTESIAN_POINT ( 'NONE',  ( 32.97430361024782997, -56.32704560409237615, -2.799357392884137763 ) ) ;
#5551=CARTESIAN_POINT ( 'NONE',  ( 34.91116660049384279, -47.87980016383388460, 2.732839075344419388 ) ) ;
#5566=CARTESIAN_POINT ( 'NONE',  ( 32.73322375381446392, -55.34783937825962141, 2.956317232382409621 ) ) ;
#5568=VECTOR ( 'NONE', #8603, 1000.000000000000000 ) ;
#5575=CARTESIAN_POINT ( 'NONE',  ( 25.17147204124252724, -52.24929059928630437, -4.731953141281072028 ) ) ;
#5576=CARTESIAN_POINT ( 'NONE',  ( 23.84527200824996029, -64.01730164816845559, 6.333338579777401556 ) ) ;
#5577=( GEOMETRIC_REPRESENTATION_CONTEXT ( 3 ) GLOBAL_UNCERTAINTY_ASSIGNED_CONTEXT ( ( #8290 ) ) GLOBAL_UNIT_ASSIGNED_CONTEXT ( ( #8710, #554, #2948 ) ) REPRESENTATION_CONTEXT ( 'NONE', 'WORKASPACE' ) );
#5582=AXIS2_PLACEMENT_3D ( 'NONE', #3891, #1512, #4979 ) ;
#5583=CARTESIAN_POINT ( 'NONE',  ( 8.718647472499544193, -59.64543329202603417, -1.841503290196028209 ) ) ;
#5585=CARTESIAN_POINT ( 'NONE',  ( 32.05770958210092658, -60.12777237996190394, 2.859594828286829760 ) ) ;
#5589=CARTESIAN_POINT ( 'NONE',  ( 18.03113812440135888, -82.24929059928629727, 4.472107801411127959 ) ) ;
#5591=EDGE_CURVE ( 'NONE', #11986, #13749, #13596, .T. ) ;
#5592=CARTESIAN_POINT ( 'NONE',  ( -12.09280073291247781, -85.24929059928631148, 11.78977872328357357 ) ) ;
#5595=CARTESIAN_POINT ( 'NONE',  ( 17.45100281819102150, -72.28366650270582738, -6.113054590618521189 ) ) ;
#5609=CARTESIAN_POINT ( 'NONE',  ( 8.094331618521831473, -56.86646964060154374, -2.513983171437783604 ) ) ;
#5617=CARTESIAN_POINT ( 'NONE',  ( 33.52366768382368889, -57.47994873761392398, 2.501453769636590607 ) ) ;
#5632=CARTESIAN_POINT ( 'NONE',  ( 29.07090146761346716, -50.97757525703124770, 4.214488946663996316 ) ) ;
#5634=DIRECTION ( 'NONE',  ( 0.000000000000000000, 0.000000000000000000, 1.000000000000000000 ) ) ;
#5637=CARTESIAN_POINT ( 'NONE',  ( 23.69232253801245847, -96.56299909827106376, -4.472107801411124406 ) ) ;
#5641=DIRECTION ( 'NONE',  ( 0.000000000000000000, 0.000000000000000000, -1.000000000000000000 ) ) ;
#5645=CARTESIAN_POINT ( 'NONE',  ( 32.50986371286720100, -54.90226484923775274, 3.064913166935400834 ) ) ;
#5655=EDGE_CURVE ( 'NONE', #7432, #9444, #14680, .T. ) ;
#5657=CARTESIAN_POINT ( 'NONE',  ( 12.08975733950408404, -52.24929059928630437, 3.124130263553816622 ) ) ;
#5659=EDGE_CURVE ( 'NONE', #1111, #4753, #967, .T. ) ;
#5664=CARTESIAN_POINT ( 'NONE',  ( 8.466388912403534306, -58.63671304798791084, -1.826958385055450274 ) ) ;
#5667=CARTESIAN_POINT ( 'NONE',  ( 33.59228746836564738, -55.86290318049214676, -1.891314907874631190 ) ) ;
#5673=CARTESIAN_POINT ( 'NONE',  ( 6.812294061964305314, -47.87980016388318205, -2.732839075317959665 ) ) ;
#5675=CARTESIAN_POINT ( 'NONE',  ( 32.90197589884652274, -57.33450387999030795, -2.749014434309867916 ) ) ;
#5678=ADVANCED_FACE ( 'NONE', ( #3594 ), #7258, .T. ) ;
#5679=CARTESIAN_POINT ( 'NONE',  ( 17.61519226005271577, -69.39711819508866597, -6.201611931792120558 ) ) ;
#5686=CARTESIAN_POINT ( 'NONE',  ( 9.937529291673584453, -54.06014836395547007, -3.368555242453570298 ) ) ;
#5704=EDGE_CURVE ( 'NONE', #9231, #10222, #797, .T. ) ;
#5711=CARTESIAN_POINT ( 'NONE',  ( 33.47544102892946682, -55.36884115291557862, -1.950692953653574424 ) ) ;
#5713=CARTESIAN_POINT ( 'NONE',  ( 23.47466359740176500, -53.10810670090260288, 6.494041865157049287 ) ) ;
#5714=ORIENTED_EDGE ( 'NONE', *, *, #14074, .T. ) ;
#5723=ADVANCED_FACE ( 'NONE', ( #3815 ), #432, .T. ) ;
#5735=CARTESIAN_POINT ( 'NONE',  ( 31.50836116271761611, -53.84182990103198563, 3.477143273224470033 ) ) ;
#5737=CARTESIAN_POINT ( 'NONE',  ( 31.49298359385885959, -60.71197230342421136, -3.050751728647420613 ) ) ;
#5746=ORIENTED_EDGE ( 'NONE', *, *, #13590, .T. ) ;
#5750=LINE ( 'NONE', #9355, #4964 ) ;
#5765=ORIENTED_EDGE ( 'NONE', *, *, #10927, .T. ) ;
#5768=CARTESIAN_POINT ( 'NONE',  ( 14.46727374856419246, -52.24929059928630437, -3.946674197044196752 ) ) ;
#5772=CARTESIAN_POINT ( 'NONE',  ( 8.903297316361205915, -55.58238924893039012, -2.909054338253188376 ) ) ;
#5786=( BOUNDED_SURFACE ( )  B_SPLINE_SURFACE ( 3, 2, ( 
 ( #6064, #14377, #9695 ),
 ( #10755, #1517, #4905 ),
 ( #2524, #6223, #7138 ),
 ( #6146, #9610, #13142 ),
 ( #5058, #2444, #7444 ),
 ( #14293, #2594, #8521 ),
 ( #7285, #14448, #10914 ),
 ( #14146, #7366, #1442 ),
 ( #12134, #10829, #3818 ),
 ( #1591, #13219, #9535 ),
 ( #10681, #3595, #8302 ),
 ( #12998, #11825, #289 ),
 ( #1283, #139, #14222 ),
 ( #3673, #8374, #13507 ),
 ( #6428, #9972, #14811 ),
 ( #13423, #11124, #7818 ),
 ( #3116, #8729, #10125 ),
 ( #4184, #14655, #4261 ),
 ( #7587, #1953, #8963 ),
 ( #8664, #7739, #13359 ),
 ( #2817, #12504, #13658 ),
 ( #14585, #581, #1732 ),
 ( #6650, #2888, #12278 ),
 ( #5351, #2972, #5280 ) ),
 .UNSPECIFIED., .F., .F., .F. ) 
 B_SPLINE_SURFACE_WITH_KNOTS ( ( 4, 2, 2, 2, 2, 2, 2, 2, 2, 2, 2, 4 ),
 ( 3, 3 ),
 ( 0.000000000000000000, 0.0007560557787111725275, 0.001512111557422345055, 0.001890139446777931373, 0.002268167336133517474, 0.003024223114844690110, 0.003402251004200276645, 0.003780278893555862746, 0.004158306782911448847, 0.004536334672267034948, 0.005292390450978207150, 0.006048446229689380220 ),
 ( 0.000000000000000000, 1.000000000000000000 ),
 .UNSPECIFIED. ) 
 GEOMETRIC_REPRESENTATION_ITEM ( )  RATIONAL_B_SPLINE_SURFACE ( (
 ( 1.000000000000000000, 0.8250833044923668869, 1.000000000000000000),
 ( 1.000000000000000000, 0.8244629924933065679, 1.000000000000000000),
 ( 1.000000000000000000, 0.8228453557282220387, 1.000000000000000000),
 ( 1.000000000000000000, 0.8179470878185581828, 1.000000000000000000),
 ( 1.000000000000000000, 0.8146336382298446921, 1.000000000000000000),
 ( 1.000000000000000000, 0.8088012687532375455, 1.000000000000000000),
 ( 1.000000000000000000, 0.8067039814524714636, 1.000000000000000000),
 ( 1.000000000000000000, 0.8022097056812382831, 1.000000000000000000),
 ( 1.000000000000000000, 0.7997977307760424370, 1.000000000000000000),
 ( 1.000000000000000000, 0.7922670365022502770, 1.000000000000000000),
 ( 1.000000000000000000, 0.7868330064135669044, 1.000000000000000000),
 ( 1.000000000000000000, 0.7779933494261681570, 1.000000000000000000),
 ( 1.000000000000000000, 0.7749217965224801663, 1.000000000000000000),
 ( 1.000000000000000000, 0.7686646892563575584, 1.000000000000000000),
 ( 1.000000000000000000, 0.7654626812325411311, 1.000000000000000000),
 ( 1.000000000000000000, 0.7588889951603841055, 1.000000000000000000),
 ( 1.000000000000000000, 0.7555173610300115472, 1.000000000000000000),
 ( 1.000000000000000000, 0.7485733441929113274, 1.000000000000000000),
 ( 1.000000000000000000, 0.7449916546359894864, 1.000000000000000000),
 ( 1.000000000000000000, 0.7341394734814182810, 1.000000000000000000),
 ( 1.000000000000000000, 0.7266881283995606511, 1.000000000000000000),
 ( 1.000000000000000000, 0.7111189506802885196, 1.000000000000000000),
 ( 1.000000000000000000, 0.7029851397915053424, 1.000000000000000000),
 ( 1.000000000000000000, 0.6947298545087532418, 1.000000000000000000) ) ) 
 REPRESENTATION_ITEM ( '' )  SURFACE ( )  );
#5789=CARTESIAN_POINT ( 'NONE',  ( 14.11899478931702490, -53.27035316348869998, -4.884032402486384150 ) ) ;
#5790=CARTESIAN_POINT ( 'NONE',  ( 28.02614528161576857, -65.45139068074421118, 4.123085411919490184 ) ) ;
#5800=B_SPLINE_CURVE_WITH_KNOTS ( 'NONE', 3,
 ( #3508, #9438, #5664, #3424 ),
 .UNSPECIFIED., .F., .F.,
 ( 4, 4 ),
 ( 0.000000000000000000, 0.001771943201165731641 ),
 .UNSPECIFIED. ) ;
#5803=CARTESIAN_POINT ( 'NONE',  ( 8.599030766203958009, -59.21224831720011395, 1.832439066039629916 ) ) ;
#5804=CARTESIAN_POINT ( 'NONE',  ( 28.60819688762819268, -64.14998386712014167, 4.112387283790987169 ) ) ;
#5818=LINE ( 'NONE', #6805, #4455 ) ;
#5824=DIRECTION ( 'NONE',  ( 0.000000000000000000, 0.000000000000000000, 1.000000000000000000 ) ) ;
#5825=CARTESIAN_POINT ( 'NONE',  ( 23.69232253801246557, -85.24929059928631148, -4.472107801411126182 ) ) ;
#5828=UNCERTAINTY_MEASURE_WITH_UNIT (LENGTH_MEASURE( 1.000000000000000082E-05 ), #8761, 'distance_accuracy_value', 'NONE');
#5832=VERTEX_POINT ( 'NONE', #6221 ) ;
#5833=CARTESIAN_POINT ( 'NONE',  ( 13.63626254758702849, -65.28118056119571122, -4.304032224033864651 ) ) ;
#5837=B_SPLINE_CURVE_WITH_KNOTS ( 'NONE', 3,
 ( #884, #8056, #13592, #6895 ),
 .UNSPECIFIED., .F., .F.,
 ( 4, 4 ),
 ( 0.000000000000000000, 0.0009656645577509051157 ),
 .UNSPECIFIED. ) ;
#5850=CARTESIAN_POINT ( 'NONE',  ( 24.62796245282055452, -82.24929059928629727, 1.347403282660977419 ) ) ;
#5851=ORIENTED_EDGE ( 'NONE', *, *, #13281, .T. ) ;
#5856=TOROIDAL_SURFACE ( 'NONE', #10756, 6.000000000000000000, 1.000000000000000000 ) ;
#5857=ORIENTED_EDGE ( 'NONE', *, *, #6589, .F. ) ;
#5870=DIRECTION ( 'NONE',  ( 0.000000000000000000, 1.000000000000000000, 0.000000000000000000 ) ) ;
#5872=CARTESIAN_POINT ( 'NONE',  ( 25.17147204124927029, -52.24929059928630437, 4.731953141288176568 ) ) ;
#5873=CARTESIAN_POINT ( 'NONE',  ( 27.87264666873679175, -68.05329818758237082, 4.069437918050730296 ) ) ;
#5883=ORIENTED_EDGE ( 'NONE', *, *, #13987, .T. ) ;
#5899=EDGE_CURVE ( 'NONE', #4896, #9073, #8191, .T. ) ;
#5901=CIRCLE ( 'NONE', #6613, 1.000000000000000666 ) ;
#5902=CARTESIAN_POINT ( 'NONE',  ( 33.00481318991428736, -59.64543329202602706, 1.841503290196059517 ) ) ;
#5905=B_SPLINE_CURVE_WITH_KNOTS ( 'NONE', 3,
 ( #3859, #2712, #7331, #4947, #10953, #11942, #399, #4875, #5100, #2791, #3712, #4797, #9806, #6113, #14347, #14189, #180, #7484, #3792, #12172, #8497, #13036, #9580 ),
 .UNSPECIFIED., .F., .F.,
 ( 4, 2, 2, 2, 2, 1, 2, 2, 2, 2, 2, 4 ),
 ( 3.576224061345498009E-18, 0.0009749202549226092772, 0.001949840509845214868, 0.002924760764767838674, 0.003412220892229137024, 0.003899681019690434940, 0.004387141147151732423, 0.004874601274613029472, 0.005849521529535599285, 0.006336981656996893732, 0.006824441784458187311, 0.007799362039380776206 ),
 .UNSPECIFIED. ) ;
#5907=CARTESIAN_POINT ( 'NONE',  ( 29.69047892279255763, -53.28399145779481216, 4.141535524925023637 ) ) ;
#5921=CARTESIAN_POINT ( 'NONE',  ( 8.599030766203956233, -59.21224831720010684, -1.832439066040420617 ) ) ;
#5937=EDGE_CURVE ( 'NONE', #2517, #4392, #5905, .T. ) ;
#5948=VERTEX_POINT ( 'NONE', #7861 ) ;
#5951=EDGE_CURVE ( 'NONE', #10536, #2336, #13228, .T. ) ;
#5958=CARTESIAN_POINT ( 'NONE',  ( 32.84819715060689305, -60.06858080083488005, -1.862453320359561237 ) ) ;
#5961=CARTESIAN_POINT ( 'NONE',  ( 30.84984438469776080, -61.21666426766278590, 3.284656216408393448 ) ) ;
#5962=CIRCLE ( 'NONE', #10120, 31.00000000000000000 ) ;
#5965=CARTESIAN_POINT ( 'NONE',  ( 30.63367540318802185, -53.42148821037872608, -3.802824752090919525 ) ) ;
#5970=CARTESIAN_POINT ( 'NONE',  ( 10.24895915366353272, -52.80093712146414475, -2.610064308312609604 ) ) ;
#5972=MECHANICAL_DESIGN_GEOMETRIC_PRESENTATION_REPRESENTATION('',(#11112),#8430);
#5984=CARTESIAN_POINT ( 'NONE',  ( 32.91088840096362844, -55.94973218888504363, 2.850075077558247738 ) ) ;
#5998=AXIS2_PLACEMENT_3D ( 'NONE', #383, #9783, #3696 ) ;
#6000=CARTESIAN_POINT ( 'NONE',  ( 32.52281604437752804, -59.06479067038042530, -2.757123406422443690 ) ) ;
#6004=B_SPLINE_CURVE_WITH_KNOTS ( 'NONE', 3,
 ( #2341, #9503, #7185, #14040, #10428, #11648, #5970, #3498, #6877, #10657, #11724, #6041, #9269, #3419, #2421, #8036, #3570, #10501, #8115, #14197 ),
 .UNSPECIFIED., .F., .F.,
 ( 4, 2, 2, 2, 2, 2, 2, 2, 2, 4 ),
 ( 0.000000000000000000, 0.0008540696272735388275, 0.001708139254547077655, 0.002562208881820616374, 0.003416278509094155310, 0.004270348136367694246, 0.005124417763641232748, 0.005978487390914772118, 0.006405522204551540935, 0.006832557018188310620 ),
 .UNSPECIFIED. ) ;
#6008=DIRECTION ( 'NONE',  ( 0.2245701561649796896, 0.9744137433416110161, -0.009279102705851381694 ) ) ;
#6010=CARTESIAN_POINT ( 'NONE',  ( 28.07070997989108108, -65.32322779890030517, 4.310009693574651024 ) ) ;
#6020=CARTESIAN_POINT ( 'NONE',  ( 23.10474973039556801, -52.24929059928630437, -5.564967562786268473 ) ) ;
#6024=VERTEX_POINT ( 'NONE', #3083 ) ;
#6034=CARTESIAN_POINT ( 'NONE',  ( 27.32685322894730717, -68.54652648479488164, 4.542640093672140722 ) ) ;
#6037=CARTESIAN_POINT ( 'NONE',  ( 30.30862891391975467, -52.33251913750448381, -3.960984348906268160 ) ) ;
#6040=ORIENTED_EDGE ( 'NONE', *, *, #14629, .T. ) ;
#6041=CARTESIAN_POINT ( 'NONE',  ( 8.674208537763544058, -54.35285673107798488, -2.119592934168749387 ) ) ;
#6053=CARTESIAN_POINT ( 'NONE',  ( 30.88740069622253515, -52.52081589074940382, 2.777424068827982317 ) ) ;
#6056=ORIENTED_EDGE ( 'NONE', *, *, #13504, .T. ) ;
#6064=CARTESIAN_POINT ( 'NONE',  ( 8.821484763567296383, -57.33450387999030795, 2.749014434309866584 ) ) ;
#6068=VECTOR ( 'NONE', #12073, 1000.000000000000000 ) ;
#6071=B_SPLINE_CURVE_WITH_KNOTS ( 'NONE', 3,
 ( #6786, #11477, #1935, #3330, #8026, #6556, #4319, #12728, #2177, #701 ),
 .UNSPECIFIED., .F., .F.,
 ( 4, 2, 2, 2, 4 ),
 ( 0.000000000000000000, 0.002335515930058450207, 0.004671031860116900414, 0.007006547790175350621, 0.009342063720233800828 ),
 .UNSPECIFIED. ) ;
#6075=CARTESIAN_POINT ( 'NONE',  ( 13.11297432109884653, -64.14571591460358491, 4.111538053172234974 ) ) ;
#6077=CARTESIAN_POINT ( 'NONE',  ( 29.69047892279256118, -53.28399145779480506, 4.141535524925028966 ) ) ;
#6079=VERTEX_POINT ( 'NONE', #5250 ) ;
#6087=ORIENTED_EDGE ( 'NONE', *, *, #14483, .T. ) ;
#6088=EDGE_CURVE ( 'NONE', #8692, #1292, #15072, .T. ) ;
#6094=ORIENTED_EDGE ( 'NONE', *, *, #5937, .F. ) ;
#6099=ORIENTED_EDGE ( 'NONE', *, *, #6926, .T. ) ;
#6100=CARTESIAN_POINT ( 'NONE',  ( 32.05794394608176390, -61.13769932686095387, -2.043477119560002997 ) ) ;
#6105=CIRCLE ( 'NONE', #3868, 1.000000000000000000 ) ;
#6108=CARTESIAN_POINT ( 'NONE',  ( 9.614235346878762911, -61.48375833289925652, 2.718831331508781979 ) ) ;
#6113=CARTESIAN_POINT ( 'NONE',  ( 33.12194698149885852, -54.49433873197092737, 2.092747212577964699 ) ) ;
#6114=CARTESIAN_POINT ( 'NONE',  ( 31.85020396773706608, -53.04884725814062563, -2.499854452451645503 ) ) ;
#6126=EDGE_CURVE ( 'NONE', #10908, #1089, #2780, .T. ) ;
#6129=CARTESIAN_POINT ( 'NONE',  ( 32.36593770905977152, -54.69330887924043338, 3.128542914575001888 ) ) ;
#6130=ADVANCED_FACE ( 'NONE', ( #3548 ), #3618, .T. ) ;
#6143=EDGE_CURVE ( 'NONE', #3243, #6024, #3325, .T. ) ;
#6146=CARTESIAN_POINT ( 'NONE',  ( 8.749157052166545157, -56.32704560409226247, 2.799357392884345597 ) ) ;
#6159=CARTESIAN_POINT ( 'NONE',  ( 23.47858629692699139, -53.24929059928630437, 6.492462156583989064 ) ) ;
#6173=DIRECTION ( 'NONE',  ( 0.000000000000000000, 0.000000000000000000, -1.000000000000000000 ) ) ;
#6187=CARTESIAN_POINT ( 'NONE',  ( 17.40655560130892354, -73.00063092933073960, 6.088059227066588086 ) ) ;
#6188=CARTESIAN_POINT ( 'NONE',  ( 27.86173033120691045, -69.39711819508849544, 2.500000000000000000 ) ) ;
#6191=CARTESIAN_POINT ( 'NONE',  ( 31.45192786070105129, -52.79510901551774538, -2.616251790959260859 ) ) ;
#6193=( BOUNDED_SURFACE ( )  B_SPLINE_SURFACE ( 3, 2, ( 
 ( #14934, #12707, #5713 ),
 ( #5551, #5632, #6770 ),
 ( #8171, #7009, #11697 ),
 ( #10321, #11622, #4625 ),
 ( #6932, #10401, #2079 ),
 ( #2156, #9247, #10 ),
 ( #13936, #9089, #6697 ),
 ( #2318, #9006, #6849 ),
 ( #4391, #4546, #8088 ),
 ( #920, #5790, #11536 ),
 ( #11385, #7938, #13709 ),
 ( #12552, #1155, #12791 ),
 ( #15096, #5873, #3392 ),
 ( #11457, #13778, #9320 ) ),
 .UNSPECIFIED., .F., .F., .F. ) 
 B_SPLINE_SURFACE_WITH_KNOTS ( ( 4, 2, 2, 2, 2, 2, 4 ),
 ( 3, 3 ),
 ( 0.2948322565876176915, 0.2981287057529254381, 0.3014251549182331846, 0.3080180532488486778, 0.3146109515794641709, 0.3179074007447718619, 0.3212038499100796085 ),
 ( 0.07447800286616089449, 1.000000000000000000 ),
 .UNSPECIFIED. ) 
 GEOMETRIC_REPRESENTATION_ITEM ( )  RATIONAL_B_SPLINE_SURFACE ( (
 ( 0.9996905063672956171, 0.9979222480410725460, 1.000000000000000000),
 ( 0.9996957508213679677, 0.9979574561150706957, 1.000000000000000000),
 ( 0.9997005874847066931, 0.9979899265301780398, 1.000000000000000000),
 ( 0.9997092625818482237, 0.9980481658545932167, 1.000000000000000000),
 ( 0.9997131045178146991, 0.9980739582752989891, 1.000000000000000000),
 ( 0.9997231512649209506, 0.9981414060230869856, 1.000000000000000000),
 ( 0.9997278760138150755, 0.9981731251127002880, 1.000000000000000000),
 ( 0.9997334421747796629, 0.9982104929310521291, 1.000000000000000000),
 ( 0.9997342833619660141, 0.9982161401500548870, 1.000000000000000000),
 ( 0.9997327054743884167, 0.9982055471728221718, 1.000000000000000000),
 ( 0.9997317056072283492, 0.9981988346730122919, 1.000000000000000000),
 ( 0.9997287795965361656, 0.9981791912173640924, 1.000000000000000000),
 ( 0.9997268671536081452, 0.9981663522390457066, 1.000000000000000000),
 ( 0.9997245403443034695, 0.9981507314569680878, 1.000000000000000000) ) ) 
 REPRESENTATION_ITEM ( '' )  SURFACE ( )  );
#6199=EDGE_LOOP ( 'NONE', ( #4752, #694, #300, #1851 ) ) ;
#6209=CARTESIAN_POINT ( 'NONE',  ( 27.86173033120691045, -69.39711819508849544, -3.619682905202609380 ) ) ;
#6210=CARTESIAN_POINT ( 'NONE',  ( 33.59752155145360319, -57.15949554451621140, 1.814500213260170414 ) ) ;
#6221=CARTESIAN_POINT ( 'NONE',  ( 13.86173033120691223, -69.39711819508849544, 0.000000000000000000 ) ) ;
#6223=CARTESIAN_POINT ( 'NONE',  ( 8.094283469768480899, -56.86702399164115462, 2.513921072343785479 ) ) ;
#6237=CARTESIAN_POINT ( 'NONE',  ( 29.48535251946016444, -62.76259148841293012, 3.786770376139651173 ) ) ;
#6238=EDGE_LOOP ( 'NONE', ( #5883, #5392, #2223, #11902 ) ) ;
#6242=EDGE_LOOP ( 'NONE', ( #2228, #8600, #2337, #3617 ) ) ;
#6246=CARTESIAN_POINT ( 'NONE',  ( 28.07070997989171701, -65.32322779889435083, -4.310009693574600398 ) ) ;
#6249=CARTESIAN_POINT ( 'NONE',  ( 29.35555050496136431, -52.24929059928631148, 3.199931146564417350 ) ) ;
#6260=CARTESIAN_POINT ( 'NONE',  ( 7.981381109186949097, -53.52407281587392873, 2.732083153704975675 ) ) ;
#6262=ADVANCED_FACE ( 'NONE', ( #10782 ), #13164, .T. ) ;
#6264=CARTESIAN_POINT ( 'NONE',  ( 30.16905084671320481, -53.31390540393488919, -3.970772651015822774 ) ) ;
#6268=CARTESIAN_POINT ( 'NONE',  ( 33.39134818684929940, -58.05408529505924520, -2.501672671492939148 ) ) ;
#6277=CARTESIAN_POINT ( 'NONE',  ( 23.72005712271144162, -60.79495753917990442, -6.390225278800149233 ) ) ;
#6280=CARTESIAN_POINT ( 'NONE',  ( 24.62796245282055452, -85.24929059928631148, -1.347403282660978752 ) ) ;
#6288=DIRECTION ( 'NONE',  ( -0.000000000000000000, -1.000000000000000000, -0.000000000000000000 ) ) ;
#6294=DIRECTION ( 'NONE',  ( 0.3351302520855081735, 0.000000000000000000, 0.9421718071228324387 ) ) ;
#6295=EDGE_LOOP ( 'NONE', ( #9250, #4836, #3919, #11710 ) ) ;
#6296=CARTESIAN_POINT ( 'NONE',  ( 31.49298359385885249, -60.71197230342421136, 3.050751728647400629 ) ) ;
#6303=CARTESIAN_POINT ( 'NONE',  ( 28.21768499689930465, -66.70046270226029606, -4.174231074483977011 ) ) ;
#6313=EDGE_CURVE ( 'NONE', #12307, #11741, #6965, .T. ) ;
#6315=AXIS2_PLACEMENT_3D ( 'NONE', #4082, #8567, #11096 ) ;
#6319=CARTESIAN_POINT ( 'NONE',  ( 32.85032212349066327, -60.06401564186453612, -1.862089353234912315 ) ) ;
#6325=EDGE_CURVE ( 'NONE', #10773, #7093, #8546, .T. ) ;
#6327=CARTESIAN_POINT ( 'NONE',  ( 13.81473638797212011, -67.42803803082790637, 4.083598241712443233 ) ) ;
#6332=CARTESIAN_POINT ( 'NONE',  ( 10.23047706855496486, -60.71197230342421136, -3.050751728647411731 ) ) ;
#6339=AXIS2_PLACEMENT_3D ( 'NONE', #9453, #8589, #3745 ) ;
#6345=CARTESIAN_POINT ( 'NONE',  ( 27.61655672830269381, -69.39711819508849544, -4.282389493064020058 ) ) ;
#6371=EDGE_LOOP ( 'NONE', ( #14664, #6094, #15037, #4369 ) ) ;
#6372=PRODUCT_DEFINITION ( 'UNKNOWN', '', #14446, #9213 ) ;
#6375=ORIENTED_EDGE ( 'NONE', *, *, #4142, .T. ) ;
#6386=CARTESIAN_POINT ( 'NONE',  ( 27.62809333727740224, -69.39711819508848123, 4.287213148048561351 ) ) ;
#6389=LINE ( 'NONE', #7400, #2410 ) ;
#6399=DIRECTION ( 'NONE',  ( 0.000000000000000000, 0.000000000000000000, 1.000000000000000000 ) ) ;
#6402=CYLINDRICAL_SURFACE ( 'NONE', #7363, 31.00000000000000000 ) ;
#6406=CARTESIAN_POINT ( 'NONE',  ( 8.821484763567294607, -57.33450387999030795, 2.749014434309869248 ) ) ;
#6418=DIRECTION ( 'NONE',  ( -0.000000000000000000, 1.000000000000000000, -0.000000000000000000 ) ) ;
#6427=CARTESIAN_POINT ( 'NONE',  ( 11.46205536272528036, -61.79747627231518692, 3.500139319475375821 ) ) ;
#6428=CARTESIAN_POINT ( 'NONE',  ( 9.936896301974771362, -54.06072418659005763, 3.368302239731210790 ) ) ;
#6429=CARTESIAN_POINT ( 'NONE',  ( 26.26264421955999495, -69.39711819508849544, 5.076148092048932803 ) ) ;
#6436=CARTESIAN_POINT ( 'NONE',  ( 8.848596353267785375, -60.00492685494598533, 2.531405393172750706 ) ) ;
#6440=CARTESIAN_POINT ( 'NONE',  ( 27.32034923808841498, -68.64054039872955570, 4.542265185094224833 ) ) ;
#6448=CARTESIAN_POINT ( 'NONE',  ( 31.27094208185658530, -61.76394201828218655, -3.065891788248765515 ) ) ;
#6450=CIRCLE ( 'NONE', #5226, 0.9999999999999996669 ) ;
#6462=AXIS2_PLACEMENT_3D ( 'NONE', #11978, #6288, #1363 ) ;
#6477=CARTESIAN_POINT ( 'NONE',  ( 12.23810814295215721, -62.76259148841472069, -3.786770376138867356 ) ) ;
#6479=CARTESIAN_POINT ( 'NONE',  ( 32.93458379808025427, -56.07566194134380311, 2.832314198475984757 ) ) ;
#6481=ORIENTED_EDGE ( 'NONE', *, *, #1968, .T. ) ;
#6483=CARTESIAN_POINT ( 'NONE',  ( 8.091875466796944139, -56.52532528994184702, -1.842181053809134994 ) ) ;
#6492=CARTESIAN_POINT ( 'NONE',  ( 23.93808696748097375, -66.03679020159736979, -6.288305159851794279 ) ) ;
#6496=DIRECTION ( 'NONE',  ( -0.000000000000000000, -0.000000000000000000, -1.000000000000000000 ) ) ;
#6501=CARTESIAN_POINT ( 'NONE',  ( 11.98773490706794753, -63.50313342087472535, 3.632148419028808473 ) ) ;
#6507=CARTESIAN_POINT ( 'NONE',  ( 8.599030766203952680, -59.21224831720009263, 1.832439066040497444 ) ) ;
#6509=DIRECTION ( 'NONE',  ( -0.000000000000000000, 1.000000000000000000, -0.000000000000000000 ) ) ;
#6511=CARTESIAN_POINT ( 'NONE',  ( 27.85761975137827662, -68.67486713609795856, 3.656664647229231235 ) ) ;
#6535=CIRCLE ( 'NONE', #12436, 0.9999999999999996669 ) ;
#6543=AXIS2_PLACEMENT_3D ( 'NONE', #6964, #14967, #12582 ) ;
#6556=CARTESIAN_POINT ( 'NONE',  ( 12.48148056143272733, -64.22824823034754615, 3.135769320951038441 ) ) ;
#6575=CARTESIAN_POINT ( 'NONE',  ( 31.74060458544689922, -52.97269888719504394, -2.532182285388751897 ) ) ;
#6584=ORIENTED_EDGE ( 'NONE', *, *, #8496, .F. ) ;
#6589=EDGE_CURVE ( 'NONE', #4392, #12856, #5176, .T. ) ;
#6608=ORIENTED_EDGE ( 'NONE', *, *, #3054, .T. ) ;
#6613=AXIS2_PLACEMENT_3D ( 'NONE', #8942, #8017, #6704 ) ;
#6621=EDGE_CURVE ( 'NONE', #8767, #14011, #4094, .T. ) ;
#6634=FACE_OUTER_BOUND ( 'NONE', #13314, .T. ) ;
#6640=ORIENTED_EDGE ( 'NONE', *, *, #12153, .F. ) ;
#6641=CARTESIAN_POINT ( 'NONE',  ( 13.86173033120691223, -69.39711819508849544, 3.619682905202618262 ) ) ;
#6643=DIRECTION ( 'NONE',  ( 0.000000000000000000, 1.000000000000000000, 0.000000000000000000 ) ) ;
#6647=CYLINDRICAL_SURFACE ( 'NONE', #6543, 3.999999999999999112 ) ;
#6650=CARTESIAN_POINT ( 'NONE',  ( 11.79472160519158308, -53.28554919726757078, 4.056729053556609621 ) ) ;
#6655=VERTEX_POINT ( 'NONE', #6000 ) ;
#6656=CARTESIAN_POINT ( 'NONE',  ( 9.950925458496486797, -63.13950256943069661, -2.713503986563631454 ) ) ;
#6662=CARTESIAN_POINT ( 'NONE',  ( 27.94380378979340662, -67.87804980504306229, 4.252496648647410282 ) ) ;
#6665=FACE_OUTER_BOUND ( 'NONE', #3821, .T. ) ;
#6674=CARTESIAN_POINT ( 'NONE',  ( 9.503997712277826082, -53.34604504765411548, -2.388784160331567819 ) ) ;
#6686=VECTOR ( 'NONE', #13388, 1000.000000000000000 ) ;
#6688=CARTESIAN_POINT ( 'NONE',  ( 9.841896756781917333, -61.30062302791023399, -2.840369378987436022 ) ) ;
#6697=CARTESIAN_POINT ( 'NONE',  ( 23.78962786808519780, -62.59345883553224610, 6.358786672825899267 ) ) ;
#6699=CARTESIAN_POINT ( 'NONE',  ( 33.62615711857835521, -56.24990207478605697, 2.565511669098800240 ) ) ;
#6704=DIRECTION ( 'NONE',  ( 0.9744556954135514815, -0.2245798247307444206, 0.000000000000000000 ) ) ;
#6706=CYLINDRICAL_SURFACE ( 'NONE', #2269, 31.00000000000000000 ) ;
#6711=VECTOR ( 'NONE', #3449, 1000.000000000000000 ) ;
#6715=CARTESIAN_POINT ( 'NONE',  ( 32.90197589884652274, -57.33450387999030795, 2.749014434309885235 ) ) ;
#6719=FACE_OUTER_BOUND ( 'NONE', #6238, .T. ) ;
#6731=CARTESIAN_POINT ( 'NONE',  ( 32.46549325755622561, -53.58625433320153064, -2.312436113725388154 ) ) ;
#6739=ORIENTED_EDGE ( 'NONE', *, *, #2161, .F. ) ;
#6740=CARTESIAN_POINT ( 'NONE',  ( 13.11526377478540617, -64.14998386711972955, -4.112387283790901904 ) ) ;
#6741=CARTESIAN_POINT ( 'NONE',  ( 18.24487436548682950, -53.24929059928630437, -6.492462156583989064 ) ) ;
#6744=CYLINDRICAL_SURFACE ( 'NONE', #2056, 2.000000000000000000 ) ;
#6748=CARTESIAN_POINT ( 'NONE',  ( 8.397260801138285657, -54.90543917109359029, -2.016464562560237095 ) ) ;
#6750=CARTESIAN_POINT ( 'NONE',  ( 33.25707175001029015, -58.63671304798791084, 1.826958385055428069 ) ) ;
#6754=CARTESIAN_POINT ( 'NONE',  ( 33.38971410812754215, -58.06117559053636512, 1.821720188314281286 ) ) ;
#6760=CARTESIAN_POINT ( 'NONE',  ( 20.86173033120691045, -52.24929059928630437, -3.000000000000000888 ) ) ;
#6765=FACE_OUTER_BOUND ( 'NONE', #656, .T. ) ;
#6766=DIRECTION ( 'NONE',  ( 0.000000000000000000, -1.000000000000000000, 0.000000000000000000 ) ) ;
#6770=CARTESIAN_POINT ( 'NONE',  ( 23.50212160825726215, -54.09900330344686381, 6.482993899733111576 ) ) ;
#6773=EDGE_CURVE ( 'NONE', #11741, #1508, #3129, .T. ) ;
#6781=CARTESIAN_POINT ( 'NONE',  ( 21.74884261173415467, -85.24929059928631148, 6.000000000000001776 ) ) ;
#6785=DIRECTION ( 'NONE',  ( -0.000000000000000000, -0.000000000000000000, -1.000000000000000000 ) ) ;
#6786=CARTESIAN_POINT ( 'NONE',  ( 13.86173033120691223, -69.39711819508849544, 3.619682905202618262 ) ) ;
#6794=CARTESIAN_POINT ( 'NONE',  ( 33.03201365928214273, -59.61641240690475740, 2.502824406253571610 ) ) ;
#6795=AXIS2_PLACEMENT_3D ( 'NONE', #131, #13131, #8446 ) ;
#6797=ORIENTED_EDGE ( 'NONE', *, *, #7251, .F. ) ;
#6799=CARTESIAN_POINT ( 'NONE',  ( 8.120991012190222236, -55.95216881616708804, 1.883383701763491791 ) ) ;
#6805=CARTESIAN_POINT ( 'NONE',  ( 20.86173033120691045, -52.24929059928630437, 7.000000000000000000 ) ) ;
#6807=CARTESIAN_POINT ( 'NONE',  ( 29.35555050496136431, -52.24929059928631148, -3.199931146564432449 ) ) ;
#6814=FACE_OUTER_BOUND ( 'NONE', #10396, .T. ) ;
#6815=EDGE_CURVE ( 'NONE', #5948, #14491, #14452, .T. ) ;
#6817=ORIENTED_EDGE ( 'NONE', *, *, #9886, .T. ) ;
#6828=CARTESIAN_POINT ( 'NONE',  ( 9.357522953353912598, -54.69330887924044049, -3.128542914574955702 ) ) ;
#6842=CARTESIAN_POINT ( 'NONE',  ( 10.85795585539533370, -53.50274931745887841, -3.718097397461419540 ) ) ;
#6848=CARTESIAN_POINT ( 'NONE',  ( 29.69047892279255763, -53.28399145779480506, 4.141535524925023637 ) ) ;
#6849=CARTESIAN_POINT ( 'NONE',  ( 23.93808696748067177, -66.03679020170480385, 6.288305159851943493 ) ) ;
#6851=DIRECTION ( 'NONE',  ( -1.000000000000000000, 0.000000000000000000, 0.000000000000000000 ) ) ;
#6854=ORIENTED_EDGE ( 'NONE', *, *, #684, .F. ) ;
#6871=ORIENTED_EDGE ( 'NONE', *, *, #12821, .T. ) ;
#6872=B_SPLINE_CURVE_WITH_KNOTS ( 'NONE', 3,
 ( #7570, #8869, #3035, #9889, #14573, #5186, #8715, #12264, #7727, #1861 ),
 .UNSPECIFIED., .F., .F.,
 ( 4, 2, 2, 2, 4 ),
 ( 0.000000000000000000, 0.002335515930058447605, 0.004671031860116895210, 0.007006547790175342814, 0.009342063720233790419 ),
 .UNSPECIFIED. ) ;
#6875=CARTESIAN_POINT ( 'NONE',  ( 32.18398686573303991, -61.03341231845916326, 2.731818205568650626 ) ) ;
#6877=CARTESIAN_POINT ( 'NONE',  ( 9.566432878864672418, -53.28273180918434804, -2.408293854232251174 ) ) ;
#6889=CARTESIAN_POINT ( 'NONE',  ( 10.23047706855496841, -60.71197230342421136, 3.050751728647412175 ) ) ;
#6890=CARTESIAN_POINT ( 'NONE',  ( 12.36791015745246192, -53.24929059928630437, 3.199931146564420903 ) ) ;
#6892=CARTESIAN_POINT ( 'NONE',  ( 13.25069131558226232, -58.78589452312201047, -4.200179654064304380 ) ) ;
#6895=CARTESIAN_POINT ( 'NONE',  ( 8.091875466796944139, -56.52532528994245808, 1.842181053809107238 ) ) ;
#6898=CARTESIAN_POINT ( 'NONE',  ( 27.84961282986260400, -69.39711819508849544, 3.799217554615836878 ) ) ;
#6899=DIRECTION ( 'NONE',  ( 0.000000000000000000, 0.000000000000000000, -1.000000000000000000 ) ) ;
#6901=CARTESIAN_POINT ( 'NONE',  ( 18.24487436548683306, -52.24929059928629727, -6.492462156583990840 ) ) ;
#6902=B_SPLINE_CURVE_WITH_KNOTS ( 'NONE', 3,
 ( #12885, #4941, #11634, #9486, #173, #11709, #7173, #4865, #9650, #3557 ),
 .UNSPECIFIED., .F., .F.,
 ( 4, 2, 2, 2, 4 ),
 ( 8.673617379884034509E-19, 0.002320432257317494879, 0.004640864514634988891, 0.006961296771952482469, 0.009281729029269976047 ),
 .UNSPECIFIED. ) ;
#6906=CARTESIAN_POINT ( 'NONE',  ( 9.222151644637104795, -54.90141807276702224, -3.067753764789347581 ) ) ;
#6926=EDGE_CURVE ( 'NONE', #8444, #13835, #1891, .T. ) ;
#6932=CARTESIAN_POINT ( 'NONE',  ( 34.22640527878306216, -51.17811635680435955, 2.733205671951302040 ) ) ;
#6951=CARTESIAN_POINT ( 'NONE',  ( 9.233977672013530480, -60.63235088943247320, 1.938839523630885298 ) ) ;
#6958=CARTESIAN_POINT ( 'NONE',  ( 31.72322230991231962, -61.42570632716525125, 2.132522520905399954 ) ) ;
#6960=CARTESIAN_POINT ( 'NONE',  ( 31.10334365618822261, -60.64100864355886955, 2.132522520905398622 ) ) ;
#6962=ORIENTED_EDGE ( 'NONE', *, *, #1365, .T. ) ;
#6964=CARTESIAN_POINT ( 'NONE',  ( 20.86173033120691045, -96.56299909827106376, 0.000000000000000000 ) ) ;
#6965=CIRCLE ( 'NONE', #10405, 3.999999999999999112 ) ;
#6971=CARTESIAN_POINT ( 'NONE',  ( 9.200644618036294631, -59.06479067038043240, 2.757123406423048984 ) ) ;
#6980=ORIENTED_EDGE ( 'NONE', *, *, #622, .T. ) ;
#6985=ADVANCED_FACE ( 'NONE', ( #11345 ), #15056, .F. ) ;
#6986=CARTESIAN_POINT ( 'NONE',  ( 23.63986771004770304, -58.63441909321034728, -6.426091441073434218 ) ) ;
#6988=CARTESIAN_POINT ( 'NONE',  ( 8.199792978590132009, -57.47994873761392398, -2.501453769636593716 ) ) ;
#6989=CARTESIAN_POINT ( 'NONE',  ( 10.26865515301073728, -52.78690463905002872, -2.615816816691508784 ) ) ;
#7009=CARTESIAN_POINT ( 'NONE',  ( 28.99759814586801454, -51.89519585609026109, 4.215672595248425303 ) ) ;
#7013=ORIENTED_EDGE ( 'NONE', *, *, #7991, .F. ) ;
#7018=CARTESIAN_POINT ( 'NONE',  ( 8.332112475569905641, -58.05408529505802306, 2.501672671478884169 ) ) ;
#7022=CARTESIAN_POINT ( 'NONE',  ( 33.03128477131276952, -59.61959967696117246, -2.502829331418514602 ) ) ;
#7029=EDGE_CURVE ( 'NONE', #15091, #7237, #5108, .T. ) ;
#7032=EDGE_CURVE ( 'NONE', #1828, #6079, #6105, .T. ) ;
#7033=VERTEX_POINT ( 'NONE', #10437 ) ;
#7042=CARTESIAN_POINT ( 'NONE',  ( 9.411927710346049025, -59.69665779701217190, 2.790274538705358687 ) ) ;
#7043=CARTESIAN_POINT ( 'NONE',  ( 33.18918945647200758, -54.61739641898385145, 2.842377187920258397 ) ) ;
#7045=B_SPLINE_CURVE_WITH_KNOTS ( 'NONE', 3,
 ( #14714, #1713, #13340, #14567 ),
 .UNSPECIFIED., .F., .F.,
 ( 4, 4 ),
 ( 0.000000000000000000, 0.001771943201165730340 ),
 .UNSPECIFIED. ) ;
#7049=CARTESIAN_POINT ( 'NONE',  ( 32.52281604437752804, -59.06479067038043240, 2.757123406423070744 ) ) ;
#7056=FACE_OUTER_BOUND ( 'NONE', #832, .T. ) ;
#7076=CARTESIAN_POINT ( 'NONE',  ( 14.02634622330045744, -66.46764508687286366, 4.441229594909811063 ) ) ;
#7085=CARTESIAN_POINT ( 'NONE',  ( 23.10474973039556801, -52.24929059928630437, -5.564967562786268473 ) ) ;
#7089=CARTESIAN_POINT ( 'NONE',  ( 20.86173033120691045, -53.24929059928630437, 0.000000000000000000 ) ) ;
#7093=VERTEX_POINT ( 'NONE', #9130 ) ;
#7105=CARTESIAN_POINT ( 'NONE',  ( 28.24717992610507622, -64.89641169172455193, 4.245552436241676553 ) ) ;
#7107=CARTESIAN_POINT ( 'NONE',  ( 9.200644618036294631, -59.06479067038043240, 2.757123406423048984 ) ) ;
#7108=CARTESIAN_POINT ( 'NONE',  ( 31.49680259653621306, -53.84195147944124216, -3.481029309662088789 ) ) ;
#7109=VERTEX_POINT ( 'NONE', #5825 ) ;
#7112=DIRECTION ( 'NONE',  ( -0.6198786537240976724, 0.7846976836063683791, 0.000000000000000000 ) ) ;
#7117=EDGE_CURVE ( 'NONE', #6024, #7934, #4608, .T. ) ;
#7123=ADVANCED_FACE ( 'NONE', ( #2507 ), #12558, .T. ) ;
#7124=CARTESIAN_POINT ( 'NONE',  ( 23.36173033120691400, -85.24929059928631148, -6.000000000000000888 ) ) ;
#7126=CARTESIAN_POINT ( 'NONE',  ( 14.23713579618830316, -69.39711819508849544, 4.406545790198910240 ) ) ;
#7127=CARTESIAN_POINT ( 'NONE',  ( 33.32619986127557610, -54.90543917109370398, 2.016464562562223950 ) ) ;
#7137=CARTESIAN_POINT ( 'NONE',  ( 23.47858629692700916, -53.24929059928630437, -6.492462156583981070 ) ) ;
#7138=CARTESIAN_POINT ( 'NONE',  ( 8.090312502367355663, -56.83321641073667507, 1.823854045752810960 ) ) ;
#7146=CARTESIAN_POINT ( 'NONE',  ( 38.02030736597991023, -69.39711819508849544, 2.500000000000000000 ) ) ;
#7156=AXIS2_PLACEMENT_3D ( 'NONE', #7146, #9544, #7223 ) ;
#7159=FACE_OUTER_BOUND ( 'NONE', #4496, .T. ) ;
#7161=DIRECTION ( 'NONE',  ( -0.000000000000000000, 1.000000000000000000, -0.000000000000000000 ) ) ;
#7172=FACE_OUTER_BOUND ( 'NONE', #8097, .T. ) ;
#7173=CARTESIAN_POINT ( 'NONE',  ( 28.30879605499156781, -66.31562986446991204, 3.513916789801492246 ) ) ;
#7181=AXIS2_PLACEMENT_3D ( 'NONE', #10622, #13160, #1305 ) ;
#7182=VERTEX_POINT ( 'NONE', #14625 ) ;
#7185=CARTESIAN_POINT ( 'NONE',  ( 11.81495288376024533, -52.27629750527023589, -3.048923371196201160 ) ) ;
#7186=CARTESIAN_POINT ( 'NONE',  ( 31.62070968671300975, -60.61174154192055141, -3.004298789847841267 ) ) ;
#7191=CIRCLE ( 'NONE', #4466, 2.000000000000000000 ) ;
#7199=CARTESIAN_POINT ( 'NONE',  ( 30.00655632846217102, -52.27452423507310186, 4.068013018865621611 ) ) ;
#7202=PLANE ( 'NONE',  #7299 ) ;
#7205=DIRECTION ( 'NONE',  ( 0.000000000000000000, -1.000000000000000000, 0.000000000000000000 ) ) ;
#7212=CARTESIAN_POINT ( 'NONE',  ( 13.86173033120691223, -69.39711819508849544, -3.619682905202625811 ) ) ;
#7223=DIRECTION ( 'NONE',  ( -1.000000000000000000, 0.000000000000000000, 0.000000000000000000 ) ) ;
#7225=CARTESIAN_POINT ( 'NONE',  ( 14.46727374856319948, -52.24929059928630437, 3.946674197044067522 ) ) ;
#7237=VERTEX_POINT ( 'NONE', #997 ) ;
#7245=CARTESIAN_POINT ( 'NONE',  ( 8.333746554286330266, -58.06117559053658539, 1.821720188289711828 ) ) ;
#7251=EDGE_CURVE ( 'NONE', #3243, #3807, #7538, .T. ) ;
#7252=EDGE_CURVE ( 'NONE', #14923, #13766, #9045, .T. ) ;
#7255=CARTESIAN_POINT ( 'NONE',  ( 27.41706354086110053, -67.71210253279710400, 4.528315385689345440 ) ) ;
#7258=( BOUNDED_SURFACE ( )  B_SPLINE_SURFACE ( 3, 2, ( 
 ( #10529, #14066, #12921 ),
 ( #5768, #11751, #8300 ),
 ( #9220, #12764, #13988 ),
 ( #15069, #6901, #8227 ) ),
 .UNSPECIFIED., .F., .F., .F. ) 
 B_SPLINE_SURFACE_WITH_KNOTS ( ( 4, 4 ),
 ( 3, 3 ),
 ( -5.204170427930421283E-18, 0.006683255761480927717 ),
 ( 0.000000000000000000, 1.000000000000000000 ),
 .UNSPECIFIED. ) 
 GEOMETRIC_REPRESENTATION_ITEM ( )  RATIONAL_B_SPLINE_SURFACE ( (
 ( 1.000000000000000000, 0.6947298545087535748, 1.000000000000000000),
 ( 1.000000000000000000, 0.6996284196041352432, 1.000000000000000000),
 ( 1.000000000000000000, 0.7035788727800805775, 1.000000000000000000),
 ( 1.000000000000000000, 0.7071067811865502373, 1.000000000000000000) ) ) 
 REPRESENTATION_ITEM ( '' )  SURFACE ( )  );
#7263=CARTESIAN_POINT ( 'NONE',  ( 31.74060919862615293, -60.49988549795170911, -2.962481358178278512 ) ) ;
#7272=EDGE_CURVE ( 'NONE', #6079, #13863, #7489, .T. ) ;
#7273=CARTESIAN_POINT ( 'NONE',  ( 30.16594816474676222, -53.31348408104258851, 3.971884189131149157 ) ) ;
#7285=CARTESIAN_POINT ( 'NONE',  ( 8.909806966310732435, -55.58532807872911263, 2.910983838681330926 ) ) ;
#7288=ADVANCED_FACE ( 'NONE', ( #12004 ), #1616, .F. ) ;
#7291=ORIENTED_EDGE ( 'NONE', *, *, #4744, .F. ) ;
#7296=CARTESIAN_POINT ( 'NONE',  ( 32.14997420079631496, -58.98766849246937483, 1.832439066040240094 ) ) ;
#7299=AXIS2_PLACEMENT_3D ( 'NONE', #4747, #8510, #2509 ) ;
#7302=DIRECTION ( 'NONE',  ( -0.000000000000000000, -1.000000000000000000, -0.000000000000000000 ) ) ;
#7304=ORIENTED_EDGE ( 'NONE', *, *, #14674, .T. ) ;
#7305=CARTESIAN_POINT ( 'NONE',  ( 23.69232253801246912, -85.24929059928631148, 4.472107801411126182 ) ) ;
#7318=CARTESIAN_POINT ( 'NONE',  ( 33.02260275403471468, -59.65407802634348400, -1.835581805806632438 ) ) ;
#7322=FACE_OUTER_BOUND ( 'NONE', #5215, .T. ) ;
#7328=CARTESIAN_POINT ( 'NONE',  ( 32.83279110308084370, -60.05631636466448242, 1.868376189747854577 ) ) ;
#7331=CARTESIAN_POINT ( 'NONE',  ( 29.98602442760622822, -52.28438478636454789, 3.027705649770566332 ) ) ;
#7332=CARTESIAN_POINT ( 'NONE',  ( 32.67588808858498339, -55.23312247377303663, -2.984220967394245694 ) ) ;
#7335=ORIENTED_EDGE ( 'NONE', *, *, #264, .T. ) ;
#7337=CARTESIAN_POINT ( 'NONE',  ( 23.55360291105710147, -55.94205978621073427, 6.462225911923646926 ) ) ;
#7355=CARTESIAN_POINT ( 'NONE',  ( 14.38963276113425138, -69.39711819508849544, -4.502057496415714510 ) ) ;
#7360=ORIENTED_EDGE ( 'NONE', *, *, #1858, .F. ) ;
#7363=AXIS2_PLACEMENT_3D ( 'NONE', #14493, #8636, #13481 ) ;
#7365=EDGE_LOOP ( 'NONE', ( #5538, #9211, #10592, #8935 ) ) ;
#7366=CARTESIAN_POINT ( 'NONE',  ( 8.352106461623211686, -55.04126158147143144, 2.748788379872049603 ) ) ;
#7371=ORIENTED_EDGE ( 'NONE', *, *, #5659, .T. ) ;
#7386=CARTESIAN_POINT ( 'NONE',  ( 28.23010146222003058, -64.93526722763056114, -4.251815205945953302 ) ) ;
#7391=DIRECTION ( 'NONE',  ( 0.000000000000000000, 0.000000000000000000, -1.000000000000000000 ) ) ;
#7392=CARTESIAN_POINT ( 'NONE',  ( 21.74884261173415467, -85.24929059928631148, 6.000000000000001776 ) ) ;
#7400=CARTESIAN_POINT ( 'NONE',  ( 29.35555050496136431, -52.24929059928631148, 2.500000000000000000 ) ) ;
#7405=CARTESIAN_POINT ( 'NONE',  ( 12.86631187927720354, -53.69100233678929612, 4.215531945485751386 ) ) ;
#7407=CARTESIAN_POINT ( 'NONE',  ( 20.86173033120691045, -69.39711819508849544, 0.000000000000000000 ) ) ;
#7408=CARTESIAN_POINT ( 'NONE',  ( 29.66826185475808586, -52.24929059928631148, -3.114712537284251237 ) ) ;
#7413=DIRECTION ( 'NONE',  ( 0.000000000000000000, 0.000000000000000000, 1.000000000000000000 ) ) ;
#7414=ORIENTED_EDGE ( 'NONE', *, *, #5480, .T. ) ;
#7416=CARTESIAN_POINT ( 'NONE',  ( 33.12442989620986822, -59.21224831720010684, -1.832439066040426834 ) ) ;
#7418=DIRECTION ( 'NONE',  ( -0.000000000000000000, -1.000000000000000000, -0.000000000000000000 ) ) ;
#7421=AXIS2_PLACEMENT_3D ( 'NONE', #2858, #10957, #1411 ) ;
#7431=AXIS2_PLACEMENT_3D ( 'NONE', #13845, #3378, #9232 ) ;
#7432=VERTEX_POINT ( 'NONE', #14757 ) ;
#7433=CARTESIAN_POINT ( 'NONE',  ( 17.61519226005271577, -69.39711819508866597, -6.201611931792120558 ) ) ;
#7434=CARTESIAN_POINT ( 'NONE',  ( 19.97461805067967333, -85.24929059928631148, 4.000000000000001776 ) ) ;
#7439=EDGE_LOOP ( 'NONE', ( #4437, #10993, #5521, #13882 ) ) ;
#7444=CARTESIAN_POINT ( 'NONE',  ( 8.134050929208209268, -55.84353942689834582, 1.893207994801671790 ) ) ;
#7461=CIRCLE ( 'NONE', #4757, 2.000000000000000000 ) ;
#7464=ORIENTED_EDGE ( 'NONE', *, *, #11719, .F. ) ;
#7466=CARTESIAN_POINT ( 'NONE',  ( 28.79421079956400931, -63.81378734512018269, -4.043274055230903663 ) ) ;
#7476=ORIENTED_EDGE ( 'NONE', *, *, #9501, .T. ) ;
#7482=CARTESIAN_POINT ( 'NONE',  ( 18.10076659937403676, -57.98711502979269028, 6.432599168432305170 ) ) ;
#7484=CARTESIAN_POINT ( 'NONE',  ( 33.58398609825992054, -55.86841147293986864, 1.893102220090065568 ) ) ;
#7485=CARTESIAN_POINT ( 'NONE',  ( 13.77965687262189576, -67.87804980504300545, -4.252496648640687660 ) ) ;
#7489=B_SPLINE_CURVE_WITH_KNOTS ( 'NONE', 3,
 ( #4628, #9323, #8174, #12877 ),
 .UNSPECIFIED., .F., .F.,
 ( 4, 4 ),
 ( 0.000000000000000000, 0.006683255761480919911 ),
 .UNSPECIFIED. ) ;
#7500=ORIENTED_EDGE ( 'NONE', *, *, #3115, .T. ) ;
#7508=ORIENTED_EDGE ( 'NONE', *, *, #8496, .T. ) ;
#7517=CARTESIAN_POINT ( 'NONE',  ( 13.86173033120691223, -69.39711819508849544, 2.500000000000000000 ) ) ;
#7538=CIRCLE ( 'NONE', #10528, 1.000000000000000000 ) ;
#7540=ORIENTED_EDGE ( 'NONE', *, *, #1810, .F. ) ;
#7542=CARTESIAN_POINT ( 'NONE',  ( 32.35376478511743414, -60.81027516727737492, -1.970305681586464130 ) ) ;
#7550=CARTESIAN_POINT ( 'NONE',  ( 9.124894037265468327, -59.08346394662398637, 2.725125706442365292 ) ) ;
#7555=LINE ( 'NONE', #1704, #4158 ) ;
#7558=ORIENTED_EDGE ( 'NONE', *, *, #6773, .F. ) ;
#7570=CARTESIAN_POINT ( 'NONE',  ( 27.86173033120691045, -69.39711819508849544, -3.619682905202609380 ) ) ;
#7573=CARTESIAN_POINT ( 'NONE',  ( 33.43681684131585996, -55.00297582962931386, -2.730999879046705825 ) ) ;
#7580=CARTESIAN_POINT ( 'NONE',  ( 14.09536732513642932, -69.39711819508849544, -4.287213148048568456 ) ) ;
#7584=CARTESIAN_POINT ( 'NONE',  ( 10.87912556056369873, -61.22098757970047700, 3.286659897586142076 ) ) ;
#7587=CARTESIAN_POINT ( 'NONE',  ( 10.53962429902219000, -53.65556550047445228, 3.599583915703609804 ) ) ;
#7589=DIRECTION ( 'NONE',  ( 0.2245716668862471066, 0.9744202983869689749, -0.008523410314122858294 ) ) ;
#7593=CARTESIAN_POINT ( 'NONE',  ( 9.541851365446024857, -61.03551305047443520, 2.732671606846408974 ) ) ;
#7601=ADVANCED_FACE ( 'NONE', ( #2139 ), #7747, .T. ) ;
#7605=CARTESIAN_POINT ( 'NONE',  ( 30.59344312246520659, -62.42480215138119348, -2.585081138714962368 ) ) ;
#7615=ORIENTED_EDGE ( 'NONE', *, *, #12821, .F. ) ;
#7621=CARTESIAN_POINT ( 'NONE',  ( 10.23047706855496841, -60.71197230342421136, 3.050751728647412175 ) ) ;
#7623=CARTESIAN_POINT ( 'NONE',  ( 8.741688182926928619, -56.83166877439235520, -2.758334070755373624 ) ) ;
#7631=CARTESIAN_POINT ( 'NONE',  ( 13.86157779355430186, -69.45278782524461292, -3.616934341765148719 ) ) ;
#7637=CARTESIAN_POINT ( 'NONE',  ( 29.25823701260754817, -63.07964102605458123, -3.871020209143769097 ) ) ;
#7640=AXIS2_PLACEMENT_3D ( 'NONE', #11286, #743, #12377 ) ;
#7643=CARTESIAN_POINT ( 'NONE',  ( 8.989056138305015153, -55.35059346084328524, 2.955710789589967913 ) ) ;
#7644=ADVANCED_FACE ( 'NONE', ( #1134 ), #10382, .T. ) ;
#7647=CARTESIAN_POINT ( 'NONE',  ( 27.86173033120691045, -69.39711819508849544, 0.000000000000000000 ) ) ;
#7651=VERTEX_POINT ( 'NONE', #5850 ) ;
#7652=CARTESIAN_POINT ( 'NONE',  ( 23.62269406304343988, -57.98711502976567544, -6.432599168430717995 ) ) ;
#7656=CARTESIAN_POINT ( 'NONE',  ( 31.49298359385885959, -60.71197230342421136, 3.050751728647414840 ) ) ;
#7662=CARTESIAN_POINT ( 'NONE',  ( 10.23047706855497196, -60.71197230342421847, 3.050751728647392191 ) ) ;
#7664=CARTESIAN_POINT ( 'NONE',  ( 24.10826840236108737, -69.39711819508849544, 6.201611931792130328 ) ) ;
#7669=ORIENTED_EDGE ( 'NONE', *, *, #9322, .T. ) ;
#7670=FACE_OUTER_BOUND ( 'NONE', #8915, .T. ) ;
#7677=CARTESIAN_POINT ( 'NONE',  ( 10.23047706855496308, -60.71197230342421136, -3.050751728647428607 ) ) ;
#7684=CARTESIAN_POINT ( 'NONE',  ( 31.72322230991231962, -61.42570632716525125, -2.132522520905367536 ) ) ;
#7687=CARTESIAN_POINT ( 'NONE',  ( 12.36791015745245836, -52.24929059928630437, -3.199931146564425788 ) ) ;
#7712=CARTESIAN_POINT ( 'NONE',  ( 32.98163981592925609, -56.83281747056103939, 2.758293468456500808 ) ) ;
#7722=DIRECTION ( 'NONE',  ( 0.000000000000000000, 0.000000000000000000, 1.000000000000000000 ) ) ;
#7727=CARTESIAN_POINT ( 'NONE',  ( 31.13618595441765180, -61.88944072237682548, -2.366779157396530664 ) ) ;
#7734=ORIENTED_EDGE ( 'NONE', *, *, #4, .T. ) ;
#7738=CARTESIAN_POINT ( 'NONE',  ( 13.00536048170750725, -65.29678988936913697, 3.348867343496716220 ) ) ;
#7739=CARTESIAN_POINT ( 'NONE',  ( 10.55836631292224048, -52.62744651407950869, 3.653242136006523921 ) ) ;
#7740=CARTESIAN_POINT ( 'NONE',  ( 31.47081793403788552, -52.80574453025635506, -2.610796954002106762 ) ) ;
#7747=( BOUNDED_SURFACE ( )  B_SPLINE_SURFACE ( 3, 2, ( 
 ( #12614, #12855, #13843 ),
 ( #1063, #13441, #9386 ),
 ( #6754, #2302, #11760 ),
 ( #10458, #5617, #3219 ) ),
 .UNSPECIFIED., .F., .F., .F. ) 
 B_SPLINE_SURFACE_WITH_KNOTS ( ( 4, 4 ),
 ( 3, 3 ),
 ( -6.071532165918824830E-18, 0.001771943201165730774 ),
 ( 0.000000000000000000, 1.000000000000000000 ),
 .UNSPECIFIED. ) 
 GEOMETRIC_REPRESENTATION_ITEM ( )  RATIONAL_B_SPLINE_SURFACE ( (
 ( 1.000000000000000000, 0.8308543624379416404, 1.000000000000000000),
 ( 1.000000000000000000, 0.8288551047899437307, 1.000000000000000000),
 ( 1.000000000000000000, 0.8269348987755770208, 1.000000000000000000),
 ( 1.000000000000000000, 0.8250833044923663318, 1.000000000000000000) ) ) 
 REPRESENTATION_ITEM ( '' )  SURFACE ( )  );
#7748=CARTESIAN_POINT ( 'NONE',  ( 30.86690024639267804, -53.50334687180571080, -3.717581709362814291 ) ) ;
#7775=CARTESIAN_POINT ( 'NONE',  ( 9.213596949546614567, -54.90226484923774564, -3.064913166935410604 ) ) ;
#7794=VECTOR ( 'NONE', #1885, 1000.000000000000000 ) ;
#7796=CARTESIAN_POINT ( 'NONE',  ( 8.749224225583514425, -56.32723911702734654, 2.799366360498976913 ) ) ;
#7798=CARTESIAN_POINT ( 'NONE',  ( 30.17362133822251735, -53.31455134687480779, 3.969134470563519645 ) ) ;
#7802=B_SPLINE_CURVE_WITH_KNOTS ( 'NONE', 3,
 ( #5350, #720, #5583, #13656, #4417, #10198, #10280, #4337, #3188, #5425 ),
 .UNSPECIFIED., .F., .F.,
 ( 4, 2, 2, 2, 4 ),
 ( 0.000000000000000000, 0.0006693228878568692692, 0.001338645775713738538, 0.002007968663570607916, 0.002677291551427477077 ),
 .UNSPECIFIED. ) ;
#7808=ADVANCED_FACE ( 'NONE', ( #2823 ), #9842, .F. ) ;
#7813=DIRECTION ( 'NONE',  ( -0.000000000000000000, -1.000000000000000000, -0.000000000000000000 ) ) ;
#7814=EDGE_CURVE ( 'NONE', #9843, #13835, #3971, .T. ) ;
#7818=CARTESIAN_POINT ( 'NONE',  ( 9.873256694677030154, -53.04884725814041246, 2.499854452449908671 ) ) ;
#7819=CARTESIAN_POINT ( 'NONE',  ( 32.48670927670975317, -59.22992907132844920, 2.757908842764457802 ) ) ;
#7821=PRODUCT ( 'Plastic-Headed Clamping Screw', 'Plastic-Headed Clamping Screw', '', ( #4064 ) ) ;
#7827=CARTESIAN_POINT ( 'NONE',  ( 17.53865101128009130, -70.79589105110508740, -6.161139702149304398 ) ) ;
#7838=CARTESIAN_POINT ( 'NONE',  ( 8.102845986945748535, -56.17744385466403401, -1.865378520188700540 ) ) ;
#7839=CARTESIAN_POINT ( 'NONE',  ( 31.72322230991231962, -61.42570632716525125, 2.500000000000000000 ) ) ;
#7841=( BOUNDED_SURFACE ( )  B_SPLINE_SURFACE ( 3, 2, ( 
 ( #6332, #10092, #2937 ),
 ( #14777, #544, #12398 ),
 ( #11307, #8774, #4072 ),
 ( #6477, #1923, #4155 ),
 ( #5397, #3084, #688 ),
 ( #5479, #1847, #4230 ),
 ( #12473, #4008, #13624 ),
 ( #8704, #1777, #5319 ),
 ( #5170, #9949, #11086 ),
 ( #10169, #14851, #4302 ),
 ( #14623, #8933, #13331 ),
 ( #2792, #7485, #13476 ),
 ( #615, #12173, #10017 ),
 ( #1631, #474, #7631 ) ),
 .UNSPECIFIED., .F., .F., .F. ) 
 B_SPLINE_SURFACE_WITH_KNOTS ( ( 4, 2, 2, 2, 2, 2, 4 ),
 ( 3, 3 ),
 ( 0.000000000000000000, 0.002560658414910375533, 0.003840987622365563299, 0.005121316829820751065, 0.006401646037275938832, 0.007681975244731126598, 0.01024263365964150213 ),
 ( 0.000000000000000000, 1.000000000000000000 ),
 .UNSPECIFIED. ) 
 GEOMETRIC_REPRESENTATION_ITEM ( )  RATIONAL_B_SPLINE_SURFACE ( (
 ( 1.000000000000000000, 0.8053615646146053964, 1.000000000000000000),
 ( 1.000000000000000000, 0.8105996499491067153, 1.000000000000000000),
 ( 1.000000000000000000, 0.8160199193853723276, 1.000000000000000000),
 ( 1.000000000000000000, 0.8240376314735106122, 1.000000000000000000),
 ( 1.000000000000000000, 0.8266971106456151297, 1.000000000000000000),
 ( 1.000000000000000000, 0.8319110421176818537, 1.000000000000000000),
 ( 1.000000000000000000, 0.8344214672177640013, 1.000000000000000000),
 ( 1.000000000000000000, 0.8392107060239336613, 1.000000000000000000),
 ( 1.000000000000000000, 0.8414897010532279564, 1.000000000000000000),
 ( 1.000000000000000000, 0.8457750297009817286, 1.000000000000000000),
 ( 1.000000000000000000, 0.8477871175333712150, 1.000000000000000000),
 ( 1.000000000000000000, 0.8533050377660172936, 1.000000000000000000),
 ( 1.000000000000000000, 0.8561733496716913416, 1.000000000000000000),
 ( 1.000000000000000000, 0.8581891718822912685, 1.000000000000000000) ) ) 
 REPRESENTATION_ITEM ( '' )  SURFACE ( )  );
#7842=ORIENTED_EDGE ( 'NONE', *, *, #13536, .F. ) ;
#7843=B_SPLINE_CURVE_WITH_KNOTS ( 'NONE', 3,
 ( #4769, #78, #3536, #8154, #10691, #2534, #4993, #8237, #9463, #2304 ),
 .UNSPECIFIED., .F., .F.,
 ( 4, 2, 2, 2, 4 ),
 ( 0.000000000000000000, 0.0004999547661763326014, 0.0009999095323526652028, 0.001499864298528997804, 0.001999819064705330406 ),
 .UNSPECIFIED. ) ;
#7848=ORIENTED_EDGE ( 'NONE', *, *, #684, .T. ) ;
#7849=ADVANCED_FACE ( 'NONE', ( #585 ), #2871, .T. ) ;
#7851=CARTESIAN_POINT ( 'NONE',  ( 9.359011486233180577, -60.82759157437174480, -1.965556376683131212 ) ) ;
#7858=CARTESIAN_POINT ( 'NONE',  ( 27.86173033120691045, -69.39711819508849544, 3.619682905202613377 ) ) ;
#7861=CARTESIAN_POINT ( 'NONE',  ( 19.97461805067967688, -85.24929059928631148, -6.000000000000000888 ) ) ;
#7864=CARTESIAN_POINT ( 'NONE',  ( 32.96722027535705735, -56.32851134755744482, 2.801743212233187563 ) ) ;
#7871=DIRECTION ( 'NONE',  ( 0.000000000000000000, -1.000000000000000000, 0.000000000000000000 ) ) ;
#7881=CARTESIAN_POINT ( 'NONE',  ( 24.31690506110717465, -73.00063092935944553, -6.088059227065252266 ) ) ;
#7887=FACE_OUTER_BOUND ( 'NONE', #11849, .T. ) ;
#7888=CARTESIAN_POINT ( 'NONE',  ( 13.13160920566097367, -64.18054652438900121, 4.118450070759805293 ) ) ;
#7890=ADVANCED_FACE ( 'NONE', ( #7670 ), #13150, .T. ) ;
#7897=CARTESIAN_POINT ( 'NONE',  ( 7.982950795113611164, -53.52517728513006290, -2.732533236877404903 ) ) ;
#7900=CARTESIAN_POINT ( 'NONE',  ( 32.94092596975102083, -56.07151166541879661, -2.830535587930123942 ) ) ;
#7906=B_SPLINE_CURVE_WITH_KNOTS ( 'NONE', 3,
 ( #6971, #12752, #11658, #7042, #14973, #11738, #8285, #12981, #9359, #6889 ),
 .UNSPECIFIED., .F., .F.,
 ( 4, 2, 2, 2, 4 ),
 ( 0.000000000000000000, 0.0004995983118107942761, 0.0009991966236215885522, 0.001498794935432382937, 0.001998393247243177104 ),
 .UNSPECIFIED. ) ;
#7908=CARTESIAN_POINT ( 'NONE',  ( 33.52235686305655804, -57.48563641131178770, -1.816685854991392457 ) ) ;
#7909=EDGE_CURVE ( 'NONE', #14799, #8767, #2390, .T. ) ;
#7915=VECTOR ( 'NONE', #10215, 1000.000000000000000 ) ;
#7918=CARTESIAN_POINT ( 'NONE',  ( 8.760785244683058082, -54.21582538152134134, -2.947777686198771452 ) ) ;
#7930=CARTESIAN_POINT ( 'NONE',  ( 20.86173033120691045, -72.24929059928631148, 0.000000000000000000 ) ) ;
#7933=CARTESIAN_POINT ( 'NONE',  ( 33.52235686305655804, -57.48563641131178770, 1.816685854991380911 ) ) ;
#7934=VERTEX_POINT ( 'NONE', #14891 ) ;
#7937=DIRECTION ( 'NONE',  ( 0.6198786537240922323, 0.7846976836063727090, 0.000000000000000000 ) ) ;
#7938=CARTESIAN_POINT ( 'NONE',  ( 27.98508387849643242, -66.12497772677620844, 4.110792498118536642 ) ) ;
#7943=CARTESIAN_POINT ( 'NONE',  ( 33.12442989620986822, -59.21224831720011395, -1.832439066039627251 ) ) ;
#7947=EDGE_LOOP ( 'NONE', ( #3405, #13130, #2734, #1719 ) ) ;
#7952=AXIS2_PLACEMENT_3D ( 'NONE', #13000, #9456, #12768 ) ;
#7957=ADVANCED_FACE ( 'NONE', ( #6814 ), #2548, .F. ) ;
#7959=CARTESIAN_POINT ( 'NONE',  ( 32.90197589884652274, -57.33450387999030795, 2.749014434309885235 ) ) ;
#7962=CARTESIAN_POINT ( 'NONE',  ( 32.45057671215001704, -59.39518542680177404, 2.758694842812651871 ) ) ;
#7973=CARTESIAN_POINT ( 'NONE',  ( 30.60506088226031096, -52.42380682680348514, -2.856405385968803667 ) ) ;
#7979=EDGE_LOOP ( 'NONE', ( #10990, #4849 ) ) ;
#7980=CARTESIAN_POINT ( 'NONE',  ( 32.97423643683031003, -56.32723911702735364, -2.799366360498969364 ) ) ;
#7987=ORIENTED_EDGE ( 'NONE', *, *, #9818, .F. ) ;
#7989=CARTESIAN_POINT ( 'NONE',  ( 8.747270541876149608, -56.45473609427328654, -2.788978005137394689 ) ) ;
#7990=DIRECTION ( 'NONE',  ( 0.000000000000000000, 0.000000000000000000, -1.000000000000000000 ) ) ;
#7991=EDGE_CURVE ( 'NONE', #6024, #11520, #2128, .T. ) ;
#7997=CARTESIAN_POINT ( 'NONE',  ( 10.00023835250034843, -61.42570632716434176, -2.132522520905085539 ) ) ;
#8000=ADVANCED_FACE ( 'NONE', ( #2434 ), #7202, .F. ) ;
#8003=ORIENTED_EDGE ( 'NONE', *, *, #13272, .T. ) ;
#8007=CARTESIAN_POINT ( 'NONE',  ( 32.95681302906984911, -57.08478275174050509, -2.747861298826744125 ) ) ;
#8008=CARTESIAN_POINT ( 'NONE',  ( 12.03298173962126150, -53.28399145779480506, -4.141535524925039624 ) ) ;
#8017=DIRECTION ( 'NONE',  ( -0.2245701561649903200, -0.9744137433416084626, -0.009279102705857585065 ) ) ;
#8026=CARTESIAN_POINT ( 'NONE',  ( 13.15381962123460191, -65.59433601606471598, 3.409308316089458835 ) ) ;
#8035=ORIENTED_EDGE ( 'NONE', *, *, #4076, .F. ) ;
#8036=CARTESIAN_POINT ( 'NONE',  ( 8.149027651920247806, -55.81410829992091749, -1.898795180179252196 ) ) ;
#8037=CARTESIAN_POINT ( 'NONE',  ( 23.63986771004770659, -58.63441909321034018, 6.426091441073435995 ) ) ;
#8046=CARTESIAN_POINT ( 'NONE',  ( 33.32712355835607809, -54.93247203738341966, -2.014559788973314891 ) ) ;
#8047=AXIS2_PLACEMENT_3D ( 'NONE', #2064, #13840, #3296 ) ;
#8051=DIRECTION ( 'NONE',  ( 2.042496995908176064E-14, 0.000000000000000000, -1.000000000000000000 ) ) ;
#8052=EDGE_LOOP ( 'NONE', ( #11381, #89, #7734, #4770 ) ) ;
#8054=CARTESIAN_POINT ( 'NONE',  ( 8.288157001243341426, -55.00412896302379551, -2.731447707962757931 ) ) ;
#8056=CARTESIAN_POINT ( 'NONE',  ( 8.127793058700618190, -57.16753985542792549, 1.814554119516831099 ) ) ;
#8062=CARTESIAN_POINT ( 'NONE',  ( 23.96426235118329728, -66.70789582472755797, -6.276998965480673931 ) ) ;
#8064=AXIS2_PLACEMENT_3D ( 'NONE', #14051, #4742, #10356 ) ;
#8067=CARTESIAN_POINT ( 'NONE',  ( 10.43042538306565881, -53.70781053471295508, -3.558938939092199938 ) ) ;
#8087=CARTESIAN_POINT ( 'NONE',  ( 27.25618691384012138, -52.24929059928630437, 3.946674197029100384 ) ) ;
#8088=CARTESIAN_POINT ( 'NONE',  ( 24.01697609496477526, -67.68160391986639013, 6.249260988556712526 ) ) ;
#8097=EDGE_LOOP ( 'NONE', ( #5275, #8739, #11618, #10726 ) ) ;
#8113=CARTESIAN_POINT ( 'NONE',  ( 32.84656685061834480, -60.07159297390028030, 1.862767969485127573 ) ) ;
#8115=CARTESIAN_POINT ( 'NONE',  ( 8.091875466796944139, -56.38350807138599663, -1.850427664022518348 ) ) ;
#8116=CARTESIAN_POINT ( 'NONE',  ( 8.091875466796944139, -56.52532528994245808, 1.842181053809107238 ) ) ;
#8123=DIRECTION ( 'NONE',  ( 0.000000000000000000, 1.000000000000000000, 0.000000000000000000 ) ) ;
#8129=VERTEX_POINT ( 'NONE', #52 ) ;
#8139=CARTESIAN_POINT ( 'NONE',  ( 23.55360291105711212, -55.94205978621073427, -6.462225911923639821 ) ) ;
#8142=CARTESIAN_POINT ( 'NONE',  ( 8.741820846485476082, -56.83281747056007305, -2.758293468456926245 ) ) ;
#8154=CARTESIAN_POINT ( 'NONE',  ( 9.766114723250986174, -60.25982778069332824, -2.890715052751949177 ) ) ;
#8156=VERTEX_POINT ( 'NONE', #13412 ) ;
#8160=ORIENTED_EDGE ( 'NONE', *, *, #12524, .T. ) ;
#8171=CARTESIAN_POINT ( 'NONE',  ( 34.73540223981435560, -48.72530132311712237, 2.733088102166433053 ) ) ;
#8174=CARTESIAN_POINT ( 'NONE',  ( 16.55200847196253022, -52.24929059928630437, 4.731961142181928537 ) ) ;
#8187=CARTESIAN_POINT ( 'NONE',  ( 31.72322230991231962, -61.42570632716525125, -2.132522520905367092 ) ) ;
#8191=CIRCLE ( 'NONE', #12607, 7.000000000000000000 ) ;
#8201=CARTESIAN_POINT ( 'NONE',  ( 17.61519226005271577, -69.39711819508849544, 6.201611931792121446 ) ) ;
#8207=DIRECTION ( 'NONE',  ( -0.000000000000000000, -0.000000000000000000, -1.000000000000000000 ) ) ;
#8209=ADVANCED_FACE ( 'NONE', ( #9891 ), #14144, .F. ) ;
#8213=CARTESIAN_POINT ( 'NONE',  ( 14.04997225853032461, -69.39711819508849544, 4.211076768700158013 ) ) ;
#8214=CARTESIAN_POINT ( 'NONE',  ( 32.29311415220630721, -54.59388862152662369, 3.160229925968714770 ) ) ;
#8215=CIRCLE ( 'NONE', #10634, 31.00000000000000000 ) ;
#8227=CARTESIAN_POINT ( 'NONE',  ( 18.24487436548682950, -53.24929059928630437, -6.492462156583997945 ) ) ;
#8230=CARTESIAN_POINT ( 'NONE',  ( 8.332112475568445475, -58.05408529505832149, -2.501672671511202761 ) ) ;
#8233=ORIENTED_EDGE ( 'NONE', *, *, #5591, .F. ) ;
#8237=CARTESIAN_POINT ( 'NONE',  ( 9.287096315897038323, -59.39117099671924649, -2.764779704643934188 ) ) ;
#8238=ORIENTED_EDGE ( 'NONE', *, *, #1738, .T. ) ;
#8239=ORIENTED_EDGE ( 'NONE', *, *, #13085, .T. ) ;
#8243=ADVANCED_FACE ( 'NONE', ( #6719 ), #13631, .T. ) ;
#8256=ORIENTED_EDGE ( 'NONE', *, *, #6313, .T. ) ;
#8261=CARTESIAN_POINT ( 'NONE',  ( 8.821484763567292831, -57.33450387999030795, 2.749014434309880794 ) ) ;
#8264=VERTEX_POINT ( 'NONE', #6641 ) ;
#8266=CARTESIAN_POINT ( 'NONE',  ( 32.06582363241078326, -61.15506547911481050, -2.039555069692439382 ) ) ;
#8275=CARTESIAN_POINT ( 'NONE',  ( 27.86173033120691045, -69.39711819508849544, 2.500000000000000000 ) ) ;
#8278=CARTESIAN_POINT ( 'NONE',  ( 9.175559494770816116, -57.26105658658105568, 1.816685854991392013 ) ) ;
#8285=CARTESIAN_POINT ( 'NONE',  ( 9.764632533060700226, -60.25800154558400834, 2.890242835725739479 ) ) ;
#8286=CARTESIAN_POINT ( 'NONE',  ( 32.85196700223596622, -54.05847863454827262, 2.186919301701788054 ) ) ;
#8290=UNCERTAINTY_MEASURE_WITH_UNIT (LENGTH_MEASURE( 1.000000000000000082E-05 ), #8710, 'distance_accuracy_value', 'NONE');
#8291=ORIENTED_EDGE ( 'NONE', *, *, #1194, .F. ) ;
#8293=CARTESIAN_POINT ( 'NONE',  ( 16.19117549353424579, -53.25924485586082113, 5.664696970550274102 ) ) ;
#8300=CARTESIAN_POINT ( 'NONE',  ( 14.12076545371522229, -53.27034158699088806, -4.884662653952329237 ) ) ;
#8302=CARTESIAN_POINT ( 'NONE',  ( 8.863084284310778216, -54.05488119003518221, 2.185023599737856870 ) ) ;
#8316=CARTESIAN_POINT ( 'NONE',  ( 12.02094163398139237, -52.24929059928630437, 4.175384597093461103 ) ) ;
#8330=DIRECTION ( 'NONE',  ( 0.000000000000000000, 0.000000000000000000, -1.000000000000000000 ) ) ;
#8341=CARTESIAN_POINT ( 'NONE',  ( 31.74727030611957446, -60.51242536180950538, -2.958269724472593065 ) ) ;
#8342=B_SPLINE_CURVE_WITH_KNOTS ( 'NONE', 3,
 ( #12245, #13469, #7623, #611, #3307, #10162, #12785, #7775, #3228, #10233, #9167, #835, #11448, #6842, #913, #14847, #13852, #5544 ),
 .UNSPECIFIED., .F., .F.,
 ( 4, 2, 2, 2, 2, 2, 2, 2, 4 ),
 ( 0.000000000000000000, 0.0007591815323294849030, 0.001518363064658969806, 0.002277544596988454600, 0.003036726129317939612, 0.003795907661647424623, 0.004555089193976909201, 0.005314270726306394646, 0.006073452258635879224 ),
 .UNSPECIFIED. ) ;
#8347=CARTESIAN_POINT ( 'NONE',  ( 33.25220092076087752, -54.75705460292245164, -2.044066819204659602 ) ) ;
#8349=( BOUNDED_SURFACE ( )  B_SPLINE_SURFACE ( 3, 2, ( 
 ( #7684, #13376, #8825 ),
 ( #12297, #6448, #5222 ),
 ( #7605, #14602, #5073 ),
 ( #4050, #8748, #312 ),
 ( #5296, #13446, #5004 ),
 ( #3910, #2909, #7466 ),
 ( #9710, #14392, #3834 ),
 ( #8541, #2686, #7386 ),
 ( #12076, #1540, #6246 ),
 ( #8607, #2768, #12154 ),
 ( #1608, #6303, #10998 ),
 ( #5145, #9852, #9145 ),
 ( #14750, #11429, #11511 ),
 ( #11280, #4202, #4436 ) ),
 .UNSPECIFIED., .F., .F., .F. ) 
 B_SPLINE_SURFACE_WITH_KNOTS ( ( 4, 2, 2, 2, 2, 2, 4 ),
 ( 3, 3 ),
 ( 0.000000000000000000, 0.002560658414910377267, 0.003840987622365565901, 0.005121316829820754535, 0.006401646037275943169, 0.007681975244731131802, 0.01024263365964150907 ),
 ( 0.000000000000000000, 1.000000000000000000 ),
 .UNSPECIFIED. ) 
 GEOMETRIC_REPRESENTATION_ITEM ( )  RATIONAL_B_SPLINE_SURFACE ( (
 ( 1.000000000000000000, 0.8053615646146050633, 1.000000000000000000),
 ( 1.000000000000000000, 0.8105996499491056051, 1.000000000000000000),
 ( 1.000000000000000000, 0.8160199193853731048, 1.000000000000000000),
 ( 1.000000000000000000, 0.8240376314735113894, 1.000000000000000000),
 ( 1.000000000000000000, 0.8266971106456140195, 1.000000000000000000),
 ( 1.000000000000000000, 0.8319110421176807435, 1.000000000000000000),
 ( 1.000000000000000000, 0.8344214672179540715, 1.000000000000000000),
 ( 1.000000000000000000, 0.8392107060237447014, 1.000000000000000000),
 ( 1.000000000000000000, 0.8414897010533705091, 1.000000000000000000),
 ( 1.000000000000000000, 0.8457750297008398421, 1.000000000000000000),
 ( 1.000000000000000000, 0.8477871175334191767, 1.000000000000000000),
 ( 1.000000000000000000, 0.8533050377659211483, 1.000000000000000000),
 ( 1.000000000000000000, 0.8561733496717631731, 1.000000000000000000),
 ( 1.000000000000000000, 0.8581891718822901582, 1.000000000000000000) ) ) 
 REPRESENTATION_ITEM ( '' )  SURFACE ( )  );
#8364=DIRECTION ( 'NONE',  ( -0.3738365665314423159, 0.000000000000000000, -0.9274945937977119303 ) ) ;
#8369=AXIS2_PLACEMENT_3D ( 'NONE', #13479, #8633, #6399 ) ;
#8374=CARTESIAN_POINT ( 'NONE',  ( 9.329831199630714167, -53.50309148220239308, 3.187126068577730287 ) ) ;
#8378=ORIENTED_EDGE ( 'NONE', *, *, #7272, .F. ) ;
#8399=CARTESIAN_POINT ( 'NONE',  ( 27.33382790127957662, -69.39711819508849544, -4.502057496415715399 ) ) ;
#8407=CYLINDRICAL_SURFACE ( 'NONE', #3002, 4.276034690655513337 ) ;
#8416=CARTESIAN_POINT ( 'NONE',  ( 13.69672121530045139, -65.45069003753607717, 4.122770147408488128 ) ) ;
#8417=VECTOR ( 'NONE', #14630, 1000.000000000000000 ) ;
#8422=CARTESIAN_POINT ( 'NONE',  ( 30.88809549976038582, -52.51002131803713979, -3.753497227305021777 ) ) ;
#8430=( GEOMETRIC_REPRESENTATION_CONTEXT ( 3 ) GLOBAL_UNCERTAINTY_ASSIGNED_CONTEXT ( ( #5828 ) ) GLOBAL_UNIT_ASSIGNED_CONTEXT ( ( #8761, #11223, #4590 ) ) REPRESENTATION_CONTEXT ( 'NONE', 'WORKASPACE' ) );
#8432=LINE ( 'NONE', #2345, #1160 ) ;
#8443=CARTESIAN_POINT ( 'NONE',  ( 31.16597161352219558, -52.62785358159868565, 3.652922677140724605 ) ) ;
#8444=VERTEX_POINT ( 'NONE', #14268 ) ;
#8446=DIRECTION ( 'NONE',  ( 0.000000000000000000, 0.000000000000000000, 1.000000000000000000 ) ) ;
#8449=DIRECTION ( 'NONE',  ( 0.000000000000000000, 0.000000000000000000, -1.000000000000000000 ) ) ;
#8460=VECTOR ( 'NONE', #7161, 1000.000000000000000 ) ;
#8463=ORIENTED_EDGE ( 'NONE', *, *, #14674, .F. ) ;
#8466=ORIENTED_EDGE ( 'NONE', *, *, #7252, .F. ) ;
#8469=CARTESIAN_POINT ( 'NONE',  ( 29.24282639220357538, -63.10178406536851270, 3.876738539649118298 ) ) ;
#8470=ORIENTED_EDGE ( 'NONE', *, *, #3115, .F. ) ;
#8471=CARTESIAN_POINT ( 'NONE',  ( 20.86173033120691045, -52.24929059928630437, -7.000000000000000000 ) ) ;
#8483=EDGE_CURVE ( 'NONE', #9073, #13749, #14990, .T. ) ;
#8484=ORIENTED_EDGE ( 'NONE', *, *, #15200, .F. ) ;
#8485=CARTESIAN_POINT ( 'NONE',  ( 31.72322230991231962, -61.42570632716525125, -2.132522520905369312 ) ) ;
#8493=CARTESIAN_POINT ( 'NONE',  ( 18.00340353969509266, -60.79495753912624423, 6.390225278796973996 ) ) ;
#8496=EDGE_CURVE ( 'NONE', #13863, #13766, #1715, .T. ) ;
#8497=CARTESIAN_POINT ( 'NONE',  ( 33.63218978277217985, -56.84102507669816617, 1.823659438126836285 ) ) ;
#8498=CARTESIAN_POINT ( 'NONE',  ( 31.56297971567678928, -52.84914412566560316, -3.506280953151710289 ) ) ;
#8510=DIRECTION ( 'NONE',  ( 0.000000000000000000, 1.000000000000000000, 0.000000000000000000 ) ) ;
#8513=ORIENTED_EDGE ( 'NONE', *, *, #2368, .T. ) ;
#8514=CARTESIAN_POINT ( 'NONE',  ( 8.599030766203958009, -59.21224831720011395, -1.832439066039622144 ) ) ;
#8515=ORIENTED_EDGE ( 'NONE', *, *, #1131, .F. ) ;
#8520=DIRECTION ( 'NONE',  ( -0.000000000000000000, -0.000000000000000000, -1.000000000000000000 ) ) ;
#8521=CARTESIAN_POINT ( 'NONE',  ( 8.248019633484567237, -55.36884115291471176, 1.950692953654363127 ) ) ;
#8527=AXIS2_PLACEMENT_3D ( 'NONE', #1208, #14898, #12919 ) ;
#8534=CARTESIAN_POINT ( 'NONE',  ( 16.19211320117534925, -53.25924031079303234, 5.665074923594178635 ) ) ;
#8538=LINE ( 'NONE', #11991, #9443 ) ;
#8539=ORIENTED_EDGE ( 'NONE', *, *, #5899, .T. ) ;
#8541=CARTESIAN_POINT ( 'NONE',  ( 28.71810018070638648, -65.29678988936899486, -3.348867343500047333 ) ) ;
#8543=VERTEX_POINT ( 'NONE', #12174 ) ;
#8544=CARTESIAN_POINT ( 'NONE',  ( 25.18496984658902349, -69.39711819508849544, -5.637959728397561321 ) ) ;
#8546=LINE ( 'NONE', #7392, #8460 ) ;
#8551=EDGE_LOOP ( 'NONE', ( #10111, #10637, #8463, #14214 ) ) ;
#8557=FACE_OUTER_BOUND ( 'NONE', #8617, .T. ) ;
#8559=CARTESIAN_POINT ( 'NONE',  ( 32.05890019364250065, -61.13673569060787827, 2.043233430235019910 ) ) ;
#8562=CARTESIAN_POINT ( 'NONE',  ( 31.87807348626150983, -54.14081474687885276, -3.331943113775099441 ) ) ;
#8567=DIRECTION ( 'NONE',  ( 0.000000000000000000, 0.000000000000000000, 1.000000000000000000 ) ) ;
#8573=CARTESIAN_POINT ( 'NONE',  ( 29.35555050496135721, -53.24929059928630437, -3.199931146564412021 ) ) ;
#8589=DIRECTION ( 'NONE',  ( 0.000000000000000000, 1.000000000000000000, 0.000000000000000000 ) ) ;
#8600=ORIENTED_EDGE ( 'NONE', *, *, #4333, .T. ) ;
#8601=CARTESIAN_POINT ( 'NONE',  ( 29.05371116072213056, -64.60713873539394569, 3.212402267255086930 ) ) ;
#8603=DIRECTION ( 'NONE',  ( 0.000000000000000000, -1.000000000000000000, 0.000000000000000000 ) ) ;
#8607=CARTESIAN_POINT ( 'NONE',  ( 28.31271169503250107, -66.37912134691313781, -3.509717431437875845 ) ) ;
#8617=EDGE_LOOP ( 'NONE', ( #418, #5851, #3472, #9156, #14957, #10306, #14141 ) ) ;
#8624=CARTESIAN_POINT ( 'NONE',  ( 23.36173033120691400, -82.24929059928629727, 6.000000000000001776 ) ) ;
#8625=AXIS2_PLACEMENT_3D ( 'NONE', #5516, #9207, #14972 ) ;
#8627=CARTESIAN_POINT ( 'NONE',  ( 17.70648456744905275, -67.68160391992790892, 6.249260988556712526 ) ) ;
#8631=CARTESIAN_POINT ( 'NONE',  ( 32.44598258732901286, -53.56578013995665088, -2.318572182806100557 ) ) ;
#8633=DIRECTION ( 'NONE',  ( 0.000000000000000000, 1.000000000000000000, 0.000000000000000000 ) ) ;
#8636=DIRECTION ( 'NONE',  ( -0.000000000000000000, 1.000000000000000000, -0.000000000000000000 ) ) ;
#8649=CARTESIAN_POINT ( 'NONE',  ( 32.22797764705516244, -60.90019506145032580, -2.720530867584999513 ) ) ;
#8652=VERTEX_POINT ( 'NONE', #7943 ) ;
#8659=ADVANCED_FACE ( 'NONE', ( #9465 ), #4090, .T. ) ;
#8661=DIRECTION ( 'NONE',  ( -1.000000000000000000, 0.000000000000000000, 0.000000000000000000 ) ) ;
#8664=CARTESIAN_POINT ( 'NONE',  ( 10.86504213735824642, -53.50006564588471036, 3.720697674322940962 ) ) ;
#8668=EDGE_CURVE ( 'NONE', #143, #10195, #10408, .T. ) ;
#8676=AXIS2_PLACEMENT_3D ( 'NONE', #5300, #14679, #8830 ) ;
#8685=FACE_OUTER_BOUND ( 'NONE', #1743, .T. ) ;
#8689=EDGE_LOOP ( 'NONE', ( #2699, #12303, #12834, #7414 ) ) ;
#8690=VECTOR ( 'NONE', #4435, 1000.000000000000000 ) ;
#8692=VERTEX_POINT ( 'NONE', #2536 ) ;
#8700=CARTESIAN_POINT ( 'NONE',  ( 12.93430674223484012, -54.56989982945474793, 4.214561586068453991 ) ) ;
#8703=DIRECTION ( 'NONE',  ( 0.000000000000000000, 0.000000000000000000, -1.000000000000000000 ) ) ;
#8704=CARTESIAN_POINT ( 'NONE',  ( 13.49335920019348833, -64.93526722763056114, -4.251815205945797871 ) ) ;
#8709=DIRECTION ( 'NONE',  ( -0.2245716668862471899, -0.9744202983869689749, -0.008523410314122886050 ) ) ;
#8710=( LENGTH_UNIT ( ) NAMED_UNIT ( * ) SI_UNIT ( .MILLI., .METRE. ) );
#8712=CARTESIAN_POINT ( 'NONE',  ( 10.85656041602113753, -53.50334687180571791, 3.717581709362825393 ) ) ;
#8715=CARTESIAN_POINT ( 'NONE',  ( 29.66000553811799634, -63.57773214734891098, -2.964070158660720100 ) ) ;
#8716=APPLICATION_CONTEXT ( 'automotive_design' ) ;
#8718=CARTESIAN_POINT ( 'NONE',  ( 28.85714878300505504, -53.69100233675187894, -4.215531945130809532 ) ) ;
#8719=ORIENTED_EDGE ( 'NONE', *, *, #4076, .T. ) ;
#8724=CARTESIAN_POINT ( 'NONE',  ( 9.200644618036294631, -59.06479067038043240, 2.757123406423048984 ) ) ;
#8725=B_SPLINE_CURVE_WITH_KNOTS ( 'NONE', 3,
 ( #14896, #10444, #11669, #1116, #9291, #5833, #15065, #6740, #4352, #10293, #14982, #4513, #2208, #9217 ),
 .UNSPECIFIED., .F., .F.,
 ( 4, 2, 2, 2, 2, 2, 4 ),
 ( 5.333844516275199261E-16, 0.002515995007885866910, 0.003773992511828533000, 0.005031990015771198657, 0.006289987519713865181, 0.007547985023656532573, 0.01006398003154186128 ),
 .UNSPECIFIED. ) ;
#8726=B_SPLINE_CURVE_WITH_KNOTS ( 'NONE', 3,
 ( #4820, #9523, #10745, #15135 ),
 .UNSPECIFIED., .F., .F.,
 ( 4, 4 ),
 ( 0.000000000000000000, 0.001771943201165731424 ),
 .UNSPECIFIED. ) ;
#8727=DIRECTION ( 'NONE',  ( -0.7546336727145995793, -0.5961293309129263029, -0.2741493039031495660 ) ) ;
#8729=CARTESIAN_POINT ( 'NONE',  ( 9.783312177552611288, -53.10528739703777745, 3.364210193422589423 ) ) ;
#8738=CARTESIAN_POINT ( 'NONE',  ( 30.63598825987613949, -53.42215338339671149, -3.801984355195810128 ) ) ;
#8739=ORIENTED_EDGE ( 'NONE', *, *, #13638, .F. ) ;
#8745=ORIENTED_EDGE ( 'NONE', *, *, #4166, .F. ) ;
#8746=ADVANCED_FACE ( 'NONE', ( #9622 ), #12464, .T. ) ;
#8748=CARTESIAN_POINT ( 'NONE',  ( 29.96883933646627440, -63.18892729117106200, -3.546101824481814990 ) ) ;
#8751=AXIS2_PLACEMENT_3D ( 'NONE', #15215, #10527, #9293 ) ;
#8754=DIRECTION ( 'NONE',  ( -0.000000000000000000, -0.000000000000000000, -1.000000000000000000 ) ) ;
#8759=ORIENTED_EDGE ( 'NONE', *, *, #6126, .T. ) ;
#8761=( LENGTH_UNIT ( ) NAMED_UNIT ( * ) SI_UNIT ( .MILLI., .METRE. ) );
#8767=VERTEX_POINT ( 'NONE', #1678 ) ;
#8774=CARTESIAN_POINT ( 'NONE',  ( 11.00886140161535387, -62.29356353673586000, -3.270869388470717176 ) ) ;
#8785=ORIENTED_EDGE ( 'NONE', *, *, #10082, .T. ) ;
#8797=CARTESIAN_POINT ( 'NONE',  ( 23.53111059739647715, -55.08889408819338485, -6.471126372657454162 ) ) ;
#8806=CARTESIAN_POINT ( 'NONE',  ( 10.59452993935293641, -61.89517205450620452, 2.369674354353247914 ) ) ;
#8811=CARTESIAN_POINT ( 'NONE',  ( 19.97461805067967688, -85.24929059928631148, -6.000000000000000888 ) ) ;
#8813=CARTESIAN_POINT ( 'NONE',  ( 9.754844199345544808, -60.26934622950999199, 2.884867303495438851 ) ) ;
#8817=DIRECTION ( 'NONE',  ( 0.000000000000000000, 0.000000000000000000, 1.000000000000000000 ) ) ;
#8825=CARTESIAN_POINT ( 'NONE',  ( 31.49298359385885249, -60.71197230342421136, -3.050751728647392191 ) ) ;
#8830=DIRECTION ( 'NONE',  ( -1.000000000000000000, 0.000000000000000000, 0.000000000000000000 ) ) ;
#8851=CARTESIAN_POINT ( 'NONE',  ( 33.52366768382369600, -57.47994873761393109, -2.501453769636598601 ) ) ;
#8869=CARTESIAN_POINT ( 'NONE',  ( 27.86173033120691400, -68.61243380581731799, -3.657093847832743716 ) ) ;
#8871=AXIS2_PLACEMENT_3D ( 'NONE', #2076, #6766, #7391 ) ;
#8876=FACE_OUTER_BOUND ( 'NONE', #14544, .T. ) ;
#8886=CARTESIAN_POINT ( 'NONE',  ( 12.06814882730127181, -63.62021712493068293, 2.966460067265556777 ) ) ;
#8887=DIRECTION ( 'NONE',  ( 0.000000000000000000, 0.000000000000000000, -1.000000000000000000 ) ) ;
#8890=CIRCLE ( 'NONE', #4215, 2.000000000000000000 ) ;
#8915=EDGE_LOOP ( 'NONE', ( #13372, #14350, #14890, #736 ) ) ;
#8917=EDGE_LOOP ( 'NONE', ( #7669, #3445, #5330, #5208 ) ) ;
#8926=B_SPLINE_CURVE_WITH_KNOTS ( 'NONE', 3,
 ( #15112, #9261, #1250, #4642 ),
 .UNSPECIFIED., .F., .F.,
 ( 4, 4 ),
 ( 0.000000000000000000, 0.006683255761480934656 ),
 .UNSPECIFIED. ) ;
#8931=CARTESIAN_POINT ( 'NONE',  ( 33.52235686305655804, -57.48563641131178770, -1.816685854991392457 ) ) ;
#8933=CARTESIAN_POINT ( 'NONE',  ( 13.50577566551451092, -66.70046270226328033, -4.174231074487356530 ) ) ;
#8935=ORIENTED_EDGE ( 'NONE', *, *, #2063, .T. ) ;
#8938=EDGE_CURVE ( 'NONE', #7182, #9663, #8725, .T. ) ;
#8942=CARTESIAN_POINT ( 'NONE',  ( 32.14997420079630785, -58.98766849246936772, -1.832439066039620812 ) ) ;
#8944=DIRECTION ( 'NONE',  ( 0.000000000000000000, 1.000000000000000000, 0.000000000000000000 ) ) ;
#8945=ORIENTED_EDGE ( 'NONE', *, *, #5659, .F. ) ;
#8950=PLANE ( 'NONE',  #12276 ) ;
#8954=CARTESIAN_POINT ( 'NONE',  ( 24.27245784421326391, -72.28366650270577054, -6.113054590623763218 ) ) ;
#8957=FACE_OUTER_BOUND ( 'NONE', #2716, .T. ) ;
#8962=CARTESIAN_POINT ( 'NONE',  ( 12.48247979829277199, -64.27177309650438985, 3.135762038898789683 ) ) ;
#8963=CARTESIAN_POINT ( 'NONE',  ( 10.41145220107785363, -52.71989690418637764, 2.656489712860343744 ) ) ;
#8966=CARTESIAN_POINT ( 'NONE',  ( 32.54790116764300478, -57.26105658658105568, 1.816685854991386462 ) ) ;
#8982=CARTESIAN_POINT ( 'NONE',  ( 8.092697108905420933, -56.34136508318314895, -1.853100783821761466 ) ) ;
#8997=CARTESIAN_POINT ( 'NONE',  ( 33.12442989620986822, -59.21224831720011395, 2.500000000000000000 ) ) ;
#9000=ORIENTED_EDGE ( 'NONE', *, *, #10614, .F. ) ;
#9006=CARTESIAN_POINT ( 'NONE',  ( 28.25509448139003155, -61.89662211384294466, 4.174060188878190303 ) ) ;
#9013=CARTESIAN_POINT ( 'NONE',  ( 21.74884261173415467, -82.24929059928629727, 4.000000000000001776 ) ) ;
#9018=AXIS2_PLACEMENT_3D ( 'NONE', #5135, #11199, #652 ) ;
#9031=CARTESIAN_POINT ( 'NONE',  ( 32.32247376001314620, -59.70726391082581586, 2.784470044084443430 ) ) ;
#9037=EDGE_CURVE ( 'NONE', #10038, #5948, #1495, .T. ) ;
#9038=AXIS2_PLACEMENT_3D ( 'NONE', #9411, #3480, #4940 ) ;
#9039=EDGE_CURVE ( 'NONE', #7651, #12307, #14028, .T. ) ;
#9040=ORIENTED_EDGE ( 'NONE', *, *, #9039, .F. ) ;
#9042=CARTESIAN_POINT ( 'NONE',  ( 23.69232253801246912, -82.24929059928629727, 4.472107801411126182 ) ) ;
#9043=CARTESIAN_POINT ( 'NONE',  ( 14.04356807543711660, -66.53205946168905882, 4.446982897615813002 ) ) ;
#9045=CIRCLE ( 'NONE', #11455, 1.000000000000000000 ) ;
#9046=CARTESIAN_POINT ( 'NONE',  ( 29.69047892279256118, -53.28399145779480506, 4.141535524925028966 ) ) ;
#9064=CARTESIAN_POINT ( 'NONE',  ( 8.125939110960342049, -57.15949554451674430, -1.814500213265047623 ) ) ;
#9066=CARTESIAN_POINT ( 'NONE',  ( 33.52235686305655804, -57.48563641131178770, 1.816685854991380911 ) ) ;
#9068=ORIENTED_EDGE ( 'NONE', *, *, #4333, .F. ) ;
#9073=VERTEX_POINT ( 'NONE', #7647 ) ;
#9077=EDGE_LOOP ( 'NONE', ( #15214, #4750, #8759, #8470 ) ) ;
#9081=CIRCLE ( 'NONE', #2450, 2.000000000000000000 ) ;
#9083=DIRECTION ( 'NONE',  ( -0.000000000000000000, -1.000000000000000000, 0.000000000000000000 ) ) ;
#9089=CARTESIAN_POINT ( 'NONE',  ( 28.47276934682737703, -58.78589452316695940, 4.200179654085411940 ) ) ;
#9098=ORIENTED_EDGE ( 'NONE', *, *, #4821, .T. ) ;
#9103=CARTESIAN_POINT ( 'NONE',  ( 20.86173033120691045, -72.24929059928631148, 0.000000000000000000 ) ) ;
#9109=CARTESIAN_POINT ( 'NONE',  ( 8.201103799357262858, -57.48563641131178770, 1.816685854991387794 ) ) ;
#9112=CARTESIAN_POINT ( 'NONE',  ( 33.02271496681120055, -59.65359113318972106, 1.835578343527247691 ) ) ;
#9116=B_SPLINE_CURVE_WITH_KNOTS ( 'NONE', 3,
 ( #11865, #9574, #13174, #12954 ),
 .UNSPECIFIED., .F., .F.,
 ( 4, 4 ),
 ( 0.000000000000000000, 0.006642648484603327214 ),
 .UNSPECIFIED. ) ;
#9127=CARTESIAN_POINT ( 'NONE',  ( 33.63224119599625794, -56.84162434074946191, -1.823610665447297885 ) ) ;
#9130=CARTESIAN_POINT ( 'NONE',  ( 21.74884261173415467, -82.24929059928629727, 6.000000000000001776 ) ) ;
#9133=AXIS2_PLACEMENT_3D ( 'NONE', #2663, #6418, #424 ) ;
#9135=EDGE_LOOP ( 'NONE', ( #4104, #9480, #4068, #12231 ) ) ;
#9144=VERTEX_POINT ( 'NONE', #9109 ) ;
#9145=CARTESIAN_POINT ( 'NONE',  ( 27.40406279159097380, -67.79239290437253374, -4.531617596075061094 ) ) ;
#9153=CARTESIAN_POINT ( 'NONE',  ( 8.534271205941925231, -54.61739641898338959, -2.842377187921200310 ) ) ;
#9155=CARTESIAN_POINT ( 'NONE',  ( 33.12442989620986822, -59.21224831720011395, 1.832439066039631914 ) ) ;
#9156=ORIENTED_EDGE ( 'NONE', *, *, #12996, .F. ) ;
#9164=CARTESIAN_POINT ( 'NONE',  ( 8.691447003131420601, -59.61641240690491372, -2.502824406264639645 ) ) ;
#9165=DIRECTION ( 'NONE',  ( 0.000000000000000000, 1.000000000000000000, 0.000000000000000000 ) ) ;
#9167=CARTESIAN_POINT ( 'NONE',  ( 9.835064211273984114, -54.14139889408635042, -3.328424545751999197 ) ) ;
#9176=EDGE_CURVE ( 'NONE', #302, #10002, #11282, .T. ) ;
#9177=AXIS2_PLACEMENT_3D ( 'NONE', #500, #8520, #8661 ) ;
#9187=CARTESIAN_POINT ( 'NONE',  ( 33.12582565096496268, -59.20619211347770516, -2.502190571104529138 ) ) ;
#9197=CARTESIAN_POINT ( 'NONE',  ( 31.67136219134865982, -63.64501252278665788, -2.710939438195376638 ) ) ;
#9200=CARTESIAN_POINT ( 'NONE',  ( 9.783297955193184237, -53.10754952926042449, 2.473486986449628500 ) ) ;
#9207=DIRECTION ( 'NONE',  ( 0.2245701561649794398, -0.9744137433416112382, 0.009279102705852556102 ) ) ;
#9211=ORIENTED_EDGE ( 'NONE', *, *, #10079, .T. ) ;
#9212=CARTESIAN_POINT ( 'NONE',  ( 18.24879706501205590, -53.10810670090265262, -6.494041865157049287 ) ) ;
#9213=PRODUCT_DEFINITION_CONTEXT ( 'detailed design', #2511, 'design' ) ;
#9216=VERTEX_POINT ( 'NONE', #11643 ) ;
#9217=CARTESIAN_POINT ( 'NONE',  ( 10.23047706855496308, -60.71197230342421136, -3.050751728647428607 ) ) ;
#9220=CARTESIAN_POINT ( 'NONE',  ( 16.55198862119230441, -52.24929059928630437, -4.731953141225709203 ) ) ;
#9221=EDGE_LOOP ( 'NONE', ( #1653, #6871, #1318, #5714 ) ) ;
#9225=CARTESIAN_POINT ( 'NONE',  ( 11.13720975898229071, -52.41844408481635753, -2.861639392410594507 ) ) ;
#9231=VERTEX_POINT ( 'NONE', #5737 ) ;
#9232=DIRECTION ( 'NONE',  ( -0.9744556954135530358, -0.2245798247307374262, 0.000000000000000000 ) ) ;
#9245=CARTESIAN_POINT ( 'NONE',  ( 32.85051389997479276, -55.70527662866913232, -2.889323894641942392 ) ) ;
#9247=CARTESIAN_POINT ( 'NONE',  ( 28.59252212848121033, -57.14744317397804707, 4.208698379002603573 ) ) ;
#9250=ORIENTED_EDGE ( 'NONE', *, *, #2985, .F. ) ;
#9258=EDGE_CURVE ( 'NONE', #7934, #3807, #8926, .T. ) ;
#9259=LINE ( 'NONE', #15187, #5117 ) ;
#9261=CARTESIAN_POINT ( 'NONE',  ( 16.55200847196254088, -52.24929059928630437, -4.731961142181927649 ) ) ;
#9269=CARTESIAN_POINT ( 'NONE',  ( 8.536817129504960633, -54.60521069725380983, -2.069777907921884985 ) ) ;
#9270=CARTESIAN_POINT ( 'NONE',  ( 8.673423145672954249, -54.35426670300921614, 2.119310268792462537 ) ) ;
#9283=DIRECTION ( 'NONE',  ( 0.000000000000000000, -0.000000000000000000, 1.000000000000000000 ) ) ;
#9285=ORIENTED_EDGE ( 'NONE', *, *, #1130, .T. ) ;
#9287=CARTESIAN_POINT ( 'NONE',  ( 9.126247950560001598, -59.08477032955737940, -2.725562014721529369 ) ) ;
#9291=CARTESIAN_POINT ( 'NONE',  ( 13.91363567147297253, -66.07496666188166046, -4.402666029760284871 ) ) ;
#9293=DIRECTION ( 'NONE',  ( -1.000000000000000000, 0.000000000000000000, 0.000000000000000000 ) ) ;
#9295=EDGE_CURVE ( 'NONE', #14139, #13981, #13890, .T. ) ;
#9301=CARTESIAN_POINT ( 'NONE',  ( 10.84100945985316145, -52.50793004641788997, -3.755530264040476407 ) ) ;
#9314=ADVANCED_FACE ( 'NONE', ( #621 ), #468, .T. ) ;
#9318=ADVANCED_FACE ( 'NONE', ( #3025 ), #5107, .F. ) ;
#9320=CARTESIAN_POINT ( 'NONE',  ( 24.36188411769310491, -73.69234276600514022, 6.062089035220985522 ) ) ;
#9322=EDGE_CURVE ( 'NONE', #14689, #5446, #14199, .T. ) ;
#9323=CARTESIAN_POINT ( 'NONE',  ( 14.46725369622999402, -52.24929059928630437, 3.946667064627061627 ) ) ;
#9335=CARTESIAN_POINT ( 'NONE',  ( 31.49298359385885959, -60.71197230342421136, -3.050751728647391747 ) ) ;
#9336=ADVANCED_FACE ( 'NONE', ( #1710 ), #6402, .F. ) ;
#9350=CARTESIAN_POINT ( 'NONE',  ( 32.52281604437752804, -59.06479067038042530, -2.757123406422443690 ) ) ;
#9355=CARTESIAN_POINT ( 'NONE',  ( 8.091875466796944139, -56.52532528994181860, 2.500000000000000000 ) ) ;
#9359=CARTESIAN_POINT ( 'NONE',  ( 10.10275097570081293, -60.61174154192054431, 3.004298789847828388 ) ) ;
#9360=CARTESIAN_POINT ( 'NONE',  ( 31.29303527934784768, -53.70781053471390720, 3.558938939092266551 ) ) ;
#9362=CARTESIAN_POINT ( 'NONE',  ( 12.86711739434182888, -53.69151354811842936, -4.215873134475239148 ) ) ;
#9364=EDGE_CURVE ( 'NONE', #6655, #8652, #5901, .T. ) ;
#9386=CARTESIAN_POINT ( 'NONE',  ( 32.64893181227846242, -58.48798588983477487, 2.754379989677820717 ) ) ;
#9391=VECTOR ( 'NONE', #4803, 1000.000000000000000 ) ;
#9393=DIRECTION ( 'NONE',  ( -0.000000000000000000, 1.000000000000000000, -0.000000000000000000 ) ) ;
#9404=VECTOR ( 'NONE', #266, 1000.000000000000000 ) ;
#9411=CARTESIAN_POINT ( 'NONE',  ( 80.00000000000001421, -85.24929059928631148, -6.000000000000001776 ) ) ;
#9416=LINE ( 'NONE', #10717, #4814 ) ;
#9418=EDGE_CURVE ( 'NONE', #4392, #5446, #10328, .T. ) ;
#9436=EDGE_CURVE ( 'NONE', #7093, #10251, #9081, .T. ) ;
#9438=CARTESIAN_POINT ( 'NONE',  ( 8.333746545461773181, -58.06117555224668081, -1.821720187977007965 ) ) ;
#9441=CARTESIAN_POINT ( 'NONE',  ( 13.91195367430395713, -69.39711819508848123, 3.980554831151302153 ) ) ;
#9442=CARTESIAN_POINT ( 'NONE',  ( 32.28464679875084897, -53.39687877504399438, 3.230473295587693361 ) ) ;
#9443=VECTOR ( 'NONE', #13238, 1000.000000000000000 ) ;
#9444=VERTEX_POINT ( 'NONE', #3089 ) ;
#9452=CARTESIAN_POINT ( 'NONE',  ( 23.84527200824996385, -64.01730164816846980, -6.333338579777399779 ) ) ;
#9453=CARTESIAN_POINT ( 'NONE',  ( 20.86173033120691045, -52.24929059928630437, 0.000000000000000000 ) ) ;
#9456=DIRECTION ( 'NONE',  ( 0.000000000000000000, 1.000000000000000000, 0.000000000000000000 ) ) ;
#9463=CARTESIAN_POINT ( 'NONE',  ( 9.236751385704064177, -59.22992907132844920, -2.757908842764468016 ) ) ;
#9464=ORIENTED_EDGE ( 'NONE', *, *, #13244, .F. ) ;
#9465=FACE_OUTER_BOUND ( 'NONE', #10841, .T. ) ;
#9480=ORIENTED_EDGE ( 'NONE', *, *, #9258, .F. ) ;
#9482=DIRECTION ( 'NONE',  ( -0.3738365665314423159, 0.000000000000000000, 0.9274945937977119303 ) ) ;
#9485=CARTESIAN_POINT ( 'NONE',  ( 9.200644618036294631, -59.06479067038042530, 2.757123406423259038 ) ) ;
#9486=CARTESIAN_POINT ( 'NONE',  ( 29.66000553811798568, -63.57773214734889677, 2.964070158660705445 ) ) ;
#9493=CARTESIAN_POINT ( 'NONE',  ( 31.96861646306723514, -60.26934622950980724, -2.884867303495886048 ) ) ;
#9495=CARTESIAN_POINT ( 'NONE',  ( 29.25256031600680018, -63.08803683229670156, 3.873126822354365562 ) ) ;
#9497=CARTESIAN_POINT ( 'NONE',  ( 31.59592920804998073, -53.91129217357566716, -3.442845340291982303 ) ) ;
#9501=EDGE_CURVE ( 'NONE', #3720, #13863, #6535, .T. ) ;
#9503=CARTESIAN_POINT ( 'NONE',  ( 12.08912955200521822, -52.24929059928630437, -3.123959181890475278 ) ) ;
#9505=CARTESIAN_POINT ( 'NONE',  ( 18.03113812440135888, -85.24929059928631148, 4.472107801411127959 ) ) ;
#9510=EDGE_CURVE ( 'NONE', #13766, #12779, #10724, .T. ) ;
#9515=CARTESIAN_POINT ( 'NONE',  ( 32.44794091343229780, -53.56780286158647186, 2.317958153238739882 ) ) ;
#9523=CARTESIAN_POINT ( 'NONE',  ( 8.466388912403532530, -58.63671304798791084, 1.826958385055444722 ) ) ;
#9525=ORIENTED_EDGE ( 'NONE', *, *, #2396, .T. ) ;
#9535=CARTESIAN_POINT ( 'NONE',  ( 8.688475229799015764, -54.32282595323670904, 2.125007313488405991 ) ) ;
#9538=DIRECTION ( 'NONE',  ( 0.000000000000000000, 0.000000000000000000, -1.000000000000000000 ) ) ;
#9544=DIRECTION ( 'NONE',  ( -0.000000000000000000, -0.000000000000000000, -1.000000000000000000 ) ) ;
#9545=AXIS2_PLACEMENT_3D ( 'NONE', #3820, #13001, #9538 ) ;
#9546=ORIENTED_EDGE ( 'NONE', *, *, #4821, .F. ) ;
#9547=CARTESIAN_POINT ( 'NONE',  ( 30.84433510184845773, -61.22098757969700955, 3.286659897587124401 ) ) ;
#9574=CARTESIAN_POINT ( 'NONE',  ( 25.53228516887957511, -53.25924485586082113, -5.664696970550253674 ) ) ;
#9576=CARTESIAN_POINT ( 'NONE',  ( 6.810513572378962266, -47.87885576612686123, 2.732387392847887231 ) ) ;
#9580=CARTESIAN_POINT ( 'NONE',  ( 33.52235686305655804, -57.48563641131178770, 1.816685854991380911 ) ) ;
#9581=CARTESIAN_POINT ( 'NONE',  ( 31.78656436043918987, -54.06072418659015000, -3.368302239731141512 ) ) ;
#9587=LINE ( 'NONE', #15195, #9404 ) ;
#9597=DIRECTION ( 'NONE',  ( 0.9274945937977119303, 1.645879719650006166E-15, -0.3738365665314420383 ) ) ;
#9601=CARTESIAN_POINT ( 'NONE',  ( 14.11897691353965811, -53.27035328036003392, 4.884026039770247074 ) ) ;
#9610=CARTESIAN_POINT ( 'NONE',  ( 8.089025167907525571, -56.24768769701488935, 2.562823873652622542 ) ) ;
#9622=FACE_OUTER_BOUND ( 'NONE', #9833, .T. ) ;
#9649=CARTESIAN_POINT ( 'NONE',  ( 8.464703746084037306, -58.62940108252750093, 2.501915095506599407 ) ) ;
#9650=CARTESIAN_POINT ( 'NONE',  ( 27.86173033120691400, -68.61243380581734641, 3.657093847832750377 ) ) ;
#9658=DIRECTION ( 'NONE',  ( 0.000000000000000000, 1.000000000000000000, 0.000000000000000000 ) ) ;
#9663=VERTEX_POINT ( 'NONE', #7677 ) ;
#9665=CARTESIAN_POINT ( 'NONE',  ( 31.49298359385885959, -60.71197230342421136, -3.050751728647420613 ) ) ;
#9677=CARTESIAN_POINT ( 'NONE',  ( 29.35555050496136076, -52.24929059928631148, 3.199931146564416462 ) ) ;
#9687=DIRECTION ( 'NONE',  ( 0.000000000000000000, 0.000000000000000000, -1.000000000000000000 ) ) ;
#9689=B_SPLINE_CURVE_WITH_KNOTS ( 'NONE', 3,
 ( #10057, #8293, #9601, #3587 ),
 .UNSPECIFIED., .F., .F.,
 ( 4, 4 ),
 ( 0.000000000000000000, 0.006642648484603335887 ),
 .UNSPECIFIED. ) ;
#9693=ORIENTED_EDGE ( 'NONE', *, *, #55, .T. ) ;
#9695=CARTESIAN_POINT ( 'NONE',  ( 8.201103799357262858, -57.48563641131178770, 1.816685854991388682 ) ) ;
#9703=CARTESIAN_POINT ( 'NONE',  ( 13.90935834228072743, -66.06148843087628109, 4.401172203687842455 ) ) ;
#9710=CARTESIAN_POINT ( 'NONE',  ( 29.05371116072213056, -64.60713873539394569, -3.212402267258252397 ) ) ;
#9723=ORIENTED_EDGE ( 'NONE', *, *, #9418, .F. ) ;
#9724=B_SPLINE_CURVE_WITH_KNOTS ( 'NONE', 3,
 ( #12299, #1755, #2912, #13450 ),
 .UNSPECIFIED., .F., .F.,
 ( 4, 4 ),
 ( 0.000000000000000000, 0.006683255761480933789 ),
 .UNSPECIFIED. ) ;
#9727=EDGE_CURVE ( 'NONE', #12771, #2922, #10234, .T. ) ;
#9735=CARTESIAN_POINT ( 'NONE',  ( 32.05873099921245029, -53.19870790407433248, -3.318692829849283932 ) ) ;
#9736=CARTESIAN_POINT ( 'NONE',  ( 20.86173033120691045, -52.24929059928630437, 0.000000000000000000 ) ) ;
#9739=CARTESIAN_POINT ( 'NONE',  ( 32.52281604437752804, -59.06479067038041819, -2.757123406423251044 ) ) ;
#9751=CARTESIAN_POINT ( 'NONE',  ( 29.35555050496136431, -56.52532528994181860, 2.500000000000000000 ) ) ;
#9763=CARTESIAN_POINT ( 'NONE',  ( 9.573486461617509491, -58.98766849246937483, -1.832439066040240983 ) ) ;
#9771=CARTESIAN_POINT ( 'NONE',  ( 12.03298173962126327, -53.28399145779480506, 4.141535524925031631 ) ) ;
#9783=DIRECTION ( 'NONE',  ( -0.000000000000000000, 1.000000000000000000, -0.000000000000000000 ) ) ;
#9793=ORIENTED_EDGE ( 'NONE', *, *, #4861, .T. ) ;
#9800=CARTESIAN_POINT ( 'NONE',  ( 17.78537369493595932, -66.03679020171973946, 6.288305159853288195 ) ) ;
#9803=ADVANCED_FACE ( 'NONE', ( #4353 ), #11425, .T. ) ;
#9804=CARTESIAN_POINT ( 'NONE',  ( 31.72322230991231962, -61.42570632716525125, 2.132522520905362651 ) ) ;
#9806=CARTESIAN_POINT ( 'NONE',  ( 33.04176068768711616, -54.35228707169699192, 2.121495901600882750 ) ) ;
#9818=EDGE_CURVE ( 'NONE', #7033, #6024, #10600, .T. ) ;
#9819=ADVANCED_FACE ( 'NONE', ( #7056 ), #4516, .T. ) ;
#9821=CARTESIAN_POINT ( 'NONE',  ( 9.074528850133887659, -58.48798588983495250, -2.754379989677188334 ) ) ;
#9823=CARTESIAN_POINT ( 'NONE',  ( 32.86505965715682720, -57.78267463900354528, -2.727521282214311782 ) ) ;
#9832=CARTESIAN_POINT ( 'NONE',  ( 31.10334365618823327, -60.64100864355887666, -2.132522520905395513 ) ) ;
#9833=EDGE_LOOP ( 'NONE', ( #14848, #9546, #2417, #574 ) ) ;
#9842=PLANE ( 'NONE',  #12704 ) ;
#9843=VERTEX_POINT ( 'NONE', #3741 ) ;
#9852=CARTESIAN_POINT ( 'NONE',  ( 27.94380378979190382, -67.87804980504907348, -4.252496648647420052 ) ) ;
#9872=CARTESIAN_POINT ( 'NONE',  ( 13.46770580362635350, -61.89598878762631529, 4.173736770066597046 ) ) ;
#9876=AXIS2_PLACEMENT_3D ( 'NONE', #3182, #6643, #11328 ) ;
#9882=DIRECTION ( 'NONE',  ( 0.000000000000000000, 1.000000000000000000, 0.000000000000000000 ) ) ;
#9886=EDGE_CURVE ( 'NONE', #1292, #8692, #14192, .T. ) ;
#9889=CARTESIAN_POINT ( 'NONE',  ( 28.30879605499156071, -66.31562986446991204, -3.513916789801494467 ) ) ;
#9891=FACE_OUTER_BOUND ( 'NONE', #3309, .T. ) ;
#9897=CARTESIAN_POINT ( 'NONE',  ( 20.86173033120691045, -85.24929059928631148, 0.000000000000000000 ) ) ;
#9907=AXIS2_PLACEMENT_3D ( 'NONE', #15224, #1286, #7990 ) ;
#9916=CARTESIAN_POINT ( 'NONE',  ( 29.93258319667773293, -53.28557432868839072, -4.055360768045983555 ) ) ;
#9941=PLANE ( 'NONE',  #13332 ) ;
#9949=CARTESIAN_POINT ( 'NONE',  ( 13.12221348233057938, -65.57050171853553877, -4.044987206835411797 ) ) ;
#9951=CARTESIAN_POINT ( 'NONE',  ( 32.95695892024548357, -57.08411837894883689, 2.747858231243594407 ) ) ;
#9964=CARTESIAN_POINT ( 'NONE',  ( 24.14199725330118440, -70.03159917004853696, -6.184016381205399426 ) ) ;
#9966=DIRECTION ( 'NONE',  ( -8.897452667106849240E-15, 0.000000000000000000, -1.000000000000000000 ) ) ;
#9969=CARTESIAN_POINT ( 'NONE',  ( 18.03113812440135888, -85.24929059928631148, -4.472107801411128847 ) ) ;
#9972=CARTESIAN_POINT ( 'NONE',  ( 9.438059962876366171, -53.39764053564381641, 3.230171433735036679 ) ) ;
#9975=EDGE_CURVE ( 'NONE', #11986, #2378, #640, .T. ) ;
#9976=CARTESIAN_POINT ( 'NONE',  ( 27.33382790127958728, -69.39711819508849544, 4.502057496415716287 ) ) ;
#9982=CYLINDRICAL_SURFACE ( 'NONE', #13306, 3.000000000000000888 ) ;
#9996=DIRECTION ( 'NONE',  ( -0.000000000000000000, -0.000000000000000000, -1.000000000000000000 ) ) ;
#10002=VERTEX_POINT ( 'NONE', #8724 ) ;
#10003=ORIENTED_EDGE ( 'NONE', *, *, #12909, .F. ) ;
#10017=CARTESIAN_POINT ( 'NONE',  ( 13.86584091103555494, -68.67486713609660853, -3.656664647209454166 ) ) ;
#10018=ORIENTED_EDGE ( 'NONE', *, *, #12750, .F. ) ;
#10020=CARTESIAN_POINT ( 'NONE',  ( 33.52235686305655804, -57.48563641131179480, 1.816685854991386018 ) ) ;
#10038=VERTEX_POINT ( 'NONE', #9969 ) ;
#10040=ORIENTED_EDGE ( 'NONE', *, *, #2396, .F. ) ;
#10046=CARTESIAN_POINT ( 'NONE',  ( 12.48063427020851535, -63.10178406537167461, 3.876738539648132864 ) ) ;
#10053=CARTESIAN_POINT ( 'NONE',  ( 8.692175891108391284, -59.61959967696039797, 2.502829331402146806 ) ) ;
#10057=CARTESIAN_POINT ( 'NONE',  ( 18.24487436548682240, -53.24929059928630437, 6.492462156583986399 ) ) ;
#10062=CARTESIAN_POINT ( 'NONE',  ( 20.86173033120691045, -53.24929059928630437, -7.000000000000000000 ) ) ;
#10065=LINE ( 'NONE', #5530, #7915 ) ;
#10071=CARTESIAN_POINT ( 'NONE',  ( 12.05320789569630868, -52.24929059928630437, -3.114169983393155317 ) ) ;
#10079=EDGE_CURVE ( 'NONE', #9444, #7182, #5254, .T. ) ;
#10082=EDGE_CURVE ( 'NONE', #10195, #14923, #2855, .T. ) ;
#10083=FACE_OUTER_BOUND ( 'NONE', #1265, .T. ) ;
#10091=AXIS2_PLACEMENT_3D ( 'NONE', #14954, #13488, #14717 ) ;
#10092=CARTESIAN_POINT ( 'NONE',  ( 9.841896756782940514, -61.30062302791113638, -2.840369378987790405 ) ) ;
#10094=CARTESIAN_POINT ( 'NONE',  ( 33.63312968452548546, -56.40460476644664567, 2.550424528239737754 ) ) ;
#10101=DIRECTION ( 'NONE',  ( 0.000000000000000000, 0.000000000000000000, 1.000000000000000000 ) ) ;
#10111=ORIENTED_EDGE ( 'NONE', *, *, #9037, .F. ) ;
#10115=CARTESIAN_POINT ( 'NONE',  ( 8.599030766203958009, -59.21224831720011395, 2.500000000000000000 ) ) ;
#10120=AXIS2_PLACEMENT_3D ( 'NONE', #10297, #1655, #9966 ) ;
#10122=CARTESIAN_POINT ( 'NONE',  ( 11.00886140161398075, -62.29356353674197067, 3.270869388470196704 ) ) ;
#10125=CARTESIAN_POINT ( 'NONE',  ( 10.00262207546350979, -52.95955415863831206, 2.537984986062526538 ) ) ;
#10126=CARTESIAN_POINT ( 'NONE',  ( 53.81626139532630049, -96.56299909827106376, -11.78977872328356646 ) ) ;
#10127=CARTESIAN_POINT ( 'NONE',  ( 23.36173033120691400, -85.24929059928631148, 6.000000000000001776 ) ) ;
#10133=CARTESIAN_POINT ( 'NONE',  ( 8.701532050552359010, -59.65700314074787514, 1.835602613583684706 ) ) ;
#10135=CARTESIAN_POINT ( 'NONE',  ( 32.90197589884652274, -57.33450387999030795, -2.749014434309867916 ) ) ;
#10147=CARTESIAN_POINT ( 'NONE',  ( 8.248681135559976951, -55.33002571195098795, -2.691408569076727098 ) ) ;
#10151=VERTEX_POINT ( 'NONE', #15045 ) ;
#10157=AXIS2_PLACEMENT_3D ( 'NONE', #5534, #4282, #669 ) ;
#10159=CARTESIAN_POINT ( 'NONE',  ( 27.86173033120691045, -69.39711819508849544, 3.710481764567783891 ) ) ;
#10160=CARTESIAN_POINT ( 'NONE',  ( 8.850040237151072020, -60.00774340954457386, -2.531751357931705915 ) ) ;
#10162=CARTESIAN_POINT ( 'NONE',  ( 8.902686789877913398, -55.58469383501344652, -2.908670588548444513 ) ) ;
#10169=CARTESIAN_POINT ( 'NONE',  ( 13.92771027672946538, -66.12098470289652141, -4.407543342774863149 ) ) ;
#10173=ADVANCED_FACE ( 'NONE', ( #7887 ), #6647, .T. ) ;
#10184=CARTESIAN_POINT ( 'NONE',  ( 9.665516716332046343, -61.13769932686095387, 2.043477119560002997 ) ) ;
#10185=CARTESIAN_POINT ( 'NONE',  ( 20.86173033120691045, -52.24929059928630437, 0.000000000000000000 ) ) ;
#10190=CARTESIAN_POINT ( 'NONE',  ( 24.18480965114325443, -70.79589105110501634, -6.161139702144090791 ) ) ;
#10195=VERTEX_POINT ( 'NONE', #1105 ) ;
#10198=CARTESIAN_POINT ( 'NONE',  ( 9.234879212749161681, -60.63355790302721715, -1.939046661991500775 ) ) ;
#10200=CARTESIAN_POINT ( 'NONE',  ( 33.04962008503242998, -54.34759098445695713, -2.119831996268577434 ) ) ;
#10205=CARTESIAN_POINT ( 'NONE',  ( 13.73837678375945792, -66.12497772680900709, -4.110792498370603454 ) ) ;
#10209=CARTESIAN_POINT ( 'NONE',  ( 31.30135442942146540, -53.71252461569495296, -3.555803702006928635 ) ) ;
#10211=CARTESIAN_POINT ( 'NONE',  ( 27.86188286885952081, -69.45278782524461292, 3.616934341765145167 ) ) ;
#10212=DIRECTION ( 'NONE',  ( 0.000000000000000000, -1.000000000000000000, 0.000000000000000000 ) ) ;
#10215=DIRECTION ( 'NONE',  ( 0.000000000000000000, -1.000000000000000000, 0.000000000000000000 ) ) ;
#10218=CARTESIAN_POINT ( 'NONE',  ( 9.844272519834872170, -54.14181112192125767, -3.331498666157651112 ) ) ;
#10219=FACE_OUTER_BOUND ( 'NONE', #13117, .T. ) ;
#10222=VERTEX_POINT ( 'NONE', #10348 ) ;
#10229=ORIENTED_EDGE ( 'NONE', *, *, #7029, .F. ) ;
#10233=CARTESIAN_POINT ( 'NONE',  ( 9.658440193288580389, -54.31466325532910844, -3.256939328598943195 ) ) ;
#10234=CIRCLE ( 'NONE', #2614, 3.999999999999999112 ) ;
#10241=CIRCLE ( 'NONE', #12455, 7.000000000000000000 ) ;
#10251=VERTEX_POINT ( 'NONE', #9042 ) ;
#10261=CARTESIAN_POINT ( 'NONE',  ( 30.86550480701848542, -53.50274931745886420, 3.718097397461435083 ) ) ;
#10262=CARTESIAN_POINT ( 'NONE',  ( 20.86173033120691045, -82.24929059928629727, 0.000000000000000000 ) ) ;
#10273=VECTOR ( 'NONE', #2566, 1000.000000000000000 ) ;
#10280=CARTESIAN_POINT ( 'NONE',  ( 9.369121201332232474, -60.80954383512729322, -1.970170733381408024 ) ) ;
#10283=CARTESIAN_POINT ( 'NONE',  ( 31.95734593916283472, -60.25982778069333534, 2.890715052751938074 ) ) ;
#10289=CARTESIAN_POINT ( 'NONE',  ( 13.13093853397579380, -57.14744317414096031, -4.208698379210318308 ) ) ;
#10290=EDGE_LOOP ( 'NONE', ( #11747, #13243, #4289, #9098, #15162 ) ) ;
#10293=CARTESIAN_POINT ( 'NONE',  ( 12.47090034640682354, -63.08803683229641024, -3.873126822354290955 ) ) ;
#10297=CARTESIAN_POINT ( 'NONE',  ( -12.09280073291247426, -85.24929059928631148, -11.78977872328358067 ) ) ;
#10301=CARTESIAN_POINT ( 'NONE',  ( 8.821484763567296383, -57.33450387999030795, -2.749014434309872801 ) ) ;
#10306=ORIENTED_EDGE ( 'NONE', *, *, #11719, .T. ) ;
#10320=CARTESIAN_POINT ( 'NONE',  ( 16.19116130666622766, -53.25924492462442572, -5.664691252382128894 ) ) ;
#10321=CARTESIAN_POINT ( 'NONE',  ( 34.39304362052245523, -50.37435811137176955, 2.733270616923093588 ) ) ;
#10328=LINE ( 'NONE', #13786, #3426 ) ;
#10337=CARTESIAN_POINT ( 'NONE',  ( 32.06502046912525827, -54.31466325532912975, 3.256939328598943639 ) ) ;
#10338=CARTESIAN_POINT ( 'NONE',  ( 9.074525391310594102, -58.48797006926987763, 2.754379914540423524 ) ) ;
#10342=CARTESIAN_POINT ( 'NONE',  ( 27.98566521725750178, -66.12426320361456078, -4.110478850071108248 ) ) ;
#10344=CARTESIAN_POINT ( 'NONE',  ( 27.60269520869858439, -53.27034158699310495, -4.884662653952261735 ) ) ;
#10348=CARTESIAN_POINT ( 'NONE',  ( 31.72322230991231962, -61.42570632716525125, -2.132522520905369312 ) ) ;
#10355=DIRECTION ( 'NONE',  ( -1.000000000000000000, -0.000000000000000000, -0.000000000000000000 ) ) ;
#10356=DIRECTION ( 'NONE',  ( 0.000000000000000000, -0.000000000000000000, -1.000000000000000000 ) ) ;
#10358=EDGE_CURVE ( 'NONE', #9144, #13981, #8432, .T. ) ;
#10361=CARTESIAN_POINT ( 'NONE',  ( 17.93383279432269006, -62.59345883550169987, -6.358786672823088182 ) ) ;
#10365=CARTESIAN_POINT ( 'NONE',  ( 32.77533487224304309, -57.91121052158847249, -2.751677492798594749 ) ) ;
#10377=CARTESIAN_POINT ( 'NONE',  ( 9.585944920971037675, -54.40403913628145460, -3.226152465599050778 ) ) ;
#10378=CARTESIAN_POINT ( 'NONE',  ( 24.62796245282055452, -96.56299909827106376, 1.347403282660977419 ) ) ;
#10382=CYLINDRICAL_SURFACE ( 'NONE', #12213, 7.000000000000000000 ) ;
#10396=EDGE_LOOP ( 'NONE', ( #3604, #2257, #939, #12129, #13492, #2726, #7987 ) ) ;
#10399=CARTESIAN_POINT ( 'NONE',  ( 32.94091731014317048, -56.07132046089822097, -2.830553478268885481 ) ) ;
#10400=CARTESIAN_POINT ( 'NONE',  ( 29.70251902843243030, -52.24929059928630437, 4.175384597093452221 ) ) ;
#10401=CARTESIAN_POINT ( 'NONE',  ( 28.78836361348337647, -54.57042255627918337, 4.214900875688467607 ) ) ;
#10405=AXIS2_PLACEMENT_3D ( 'NONE', #13092, #14169, #8330 ) ;
#10406=CARTESIAN_POINT ( 'NONE',  ( 16.55198862119814862, -52.24929059928630437, 4.731953141213115721 ) ) ;
#10408=B_SPLINE_CURVE_WITH_KNOTS ( 'NONE', 3,
 ( #6077, #1451, #12147, #6159 ),
 .UNSPECIFIED., .F., .F.,
 ( 4, 4 ),
 ( 0.000000000000000000, 0.006642668954637880041 ),
 .UNSPECIFIED. ) ;
#10426=CARTESIAN_POINT ( 'NONE',  ( 31.77372435728965883, -63.13800426661170206, -2.713090553711066555 ) ) ;
#10428=CARTESIAN_POINT ( 'NONE',  ( 11.00828597368551698, -52.46167102156725548, -2.825639067667213844 ) ) ;
#10430=ORIENTED_EDGE ( 'NONE', *, *, #5485, .F. ) ;
#10437=CARTESIAN_POINT ( 'NONE',  ( 17.61519226005271577, -69.39711819508866597, -6.201611931792120558 ) ) ;
#10444=CARTESIAN_POINT ( 'NONE',  ( 14.39660743346648708, -68.54652648479442689, -4.542640093672132728 ) ) ;
#10453=CARTESIAN_POINT ( 'NONE',  ( 8.152528251094548040, -55.78447712832181082, -2.622266312281611000 ) ) ;
#10456=EDGE_CURVE ( 'NONE', #302, #9144, #2397, .T. ) ;
#10458=CARTESIAN_POINT ( 'NONE',  ( 33.52235686305655804, -57.48563641131178770, 1.816685854991385574 ) ) ;
#10465=DIRECTION ( 'NONE',  ( -0.9274945937977119303, 1.321628185579677547E-15, 0.3738365665314420383 ) ) ;
#10480=DIRECTION ( 'NONE',  ( -0.9274945937977119303, -3.217893291404924306E-15, -0.3738365665314420383 ) ) ;
#10493=VECTOR ( 'NONE', #7302, 1000.000000000000000 ) ;
#10496=( BOUNDED_SURFACE ( )  B_SPLINE_SURFACE ( 3, 2, ( 
 ( #14968, #14731, #7662 ),
 ( #8806, #12355, #7584 ),
 ( #4182, #10122, #6427 ),
 ( #12277, #579, #1811 ),
 ( #8886, #6501, #10046 ),
 ( #8962, #13580, #11191 ),
 ( #3046, #11337, #7888 ),
 ( #7738, #14809, #12423 ),
 ( #1874, #13735, #12502 ),
 ( #2034, #3113, #1951 ),
 ( #798, #5513, #9043 ),
 ( #12585, #4575, #4737 ),
 ( #1193, #125, #2192 ),
 ( #12745, #10508, #3575 ) ),
 .UNSPECIFIED., .F., .F., .F. ) 
 B_SPLINE_SURFACE_WITH_KNOTS ( ( 4, 2, 2, 2, 2, 2, 4 ),
 ( 3, 3 ),
 ( 0.000000000000000000, 0.002560658414910375099, 0.003840987622365562432, 0.005121316829820750198, 0.006401646037275937964, 0.007681975244731124863, 0.01024263365964150040 ),
 ( 0.000000000000000000, 1.000000000000000000 ),
 .UNSPECIFIED. ) 
 GEOMETRIC_REPRESENTATION_ITEM ( )  RATIONAL_B_SPLINE_SURFACE ( (
 ( 1.000000000000000000, 0.8053615646146036200, 1.000000000000000000),
 ( 1.000000000000000000, 0.8105996499489666052, 1.000000000000000000),
 ( 1.000000000000000000, 0.8160199193855625088, 1.000000000000000000),
 ( 1.000000000000000000, 0.8240376314734160212, 1.000000000000000000),
 ( 1.000000000000000000, 0.8266971106455908158, 1.000000000000000000),
 ( 1.000000000000000000, 0.8319110421177055015, 1.000000000000000000),
 ( 1.000000000000000000, 0.8344214672177876491, 1.000000000000000000),
 ( 1.000000000000000000, 0.8392107060239100136, 1.000000000000000000),
 ( 1.000000000000000000, 0.8414897010531573462, 1.000000000000000000),
 ( 1.000000000000000000, 0.8457750297010532270, 1.000000000000000000),
 ( 1.000000000000000000, 0.8477871175334914522, 1.000000000000000000),
 ( 1.000000000000000000, 0.8533050377657773744, 1.000000000000000000),
 ( 1.000000000000000000, 0.8561733496718711978, 1.000000000000000000),
 ( 1.000000000000000000, 0.8581891718822912685, 1.000000000000000000) ) ) 
 REPRESENTATION_ITEM ( '' )  SURFACE ( )  );
#10501=CARTESIAN_POINT ( 'NONE',  ( 8.098912479706312340, -56.24150114312890025, -1.860592018039514350 ) ) ;
#10504=ORIENTED_EDGE ( 'NONE', *, *, #174, .F. ) ;
#10508=CARTESIAN_POINT ( 'NONE',  ( 13.86142555056148851, -69.48056866272027321, 4.214447830835809761 ) ) ;
#10514=AXIS2_PLACEMENT_3D ( 'NONE', #5592, #12666, #8051 ) ;
#10516=VECTOR ( 'NONE', #4418, 1000.000000000000000 ) ;
#10517=CARTESIAN_POINT ( 'NONE',  ( 31.49780332062879040, -53.83453582474924559, 3.481203917140397230 ) ) ;
#10520=CARTESIAN_POINT ( 'NONE',  ( 18.13205847683729388, -57.03285117767155299, -6.445925775549026682 ) ) ;
#10527=DIRECTION ( 'NONE',  ( -0.000000000000000000, -0.000000000000000000, -1.000000000000000000 ) ) ;
#10528=AXIS2_PLACEMENT_3D ( 'NONE', #3238, #96, #11778 ) ;
#10529=CARTESIAN_POINT ( 'NONE',  ( 12.36791015745246369, -52.24929059928630437, -3.199931146564426232 ) ) ;
#10532=FACE_OUTER_BOUND ( 'NONE', #5, .T. ) ;
#10536=VERTEX_POINT ( 'NONE', #1572 ) ;
#10540=CARTESIAN_POINT ( 'NONE',  ( 12.22370793440460801, -62.74348037527475697, 3.781439773221460854 ) ) ;
#10550=ORIENTED_EDGE ( 'NONE', *, *, #9510, .F. ) ;
#10553=CARTESIAN_POINT ( 'NONE',  ( 23.10474973039555024, -52.24929059928630437, 5.564967562786278243 ) ) ;
#10569=CARTESIAN_POINT ( 'NONE',  ( 23.47858629692700916, -53.24929059928630437, -6.492462156583981070 ) ) ;
#10570=FACE_OUTER_BOUND ( 'NONE', #7439, .T. ) ;
#10572=CARTESIAN_POINT ( 'NONE',  ( 30.26995075049824990, -61.78874994510989183, 3.497001979624811074 ) ) ;
#10577=ORIENTED_EDGE ( 'NONE', *, *, #753, .F. ) ;
#10581=CARTESIAN_POINT ( 'NONE',  ( 32.43704918934574977, -59.38916093354929870, -2.764669745501080911 ) ) ;
#10588=PLANE ( 'NONE',  #8064 ) ;
#10589=CARTESIAN_POINT ( 'NONE',  ( 33.37897949129445863, -55.03829860714096611, 2.746682580609041580 ) ) ;
#10592=ORIENTED_EDGE ( 'NONE', *, *, #13833, .T. ) ;
#10593=CARTESIAN_POINT ( 'NONE',  ( 21.74884261173415467, -85.24929059928631148, 4.000000000000001776 ) ) ;
#10597=CARTESIAN_POINT ( 'NONE',  ( 23.10474973039556801, -53.24929059928630437, -5.564967562786270250 ) ) ;
#10600=B_SPLINE_CURVE_WITH_KNOTS ( 'NONE', 3,
 ( #5679, #2052, #15066, #4591, #3524, #6741 ),
 .UNSPECIFIED., .F., .F.,
 ( 4, 2, 4 ),
 ( 0.000000000000000000, 0.008081365602590071667, 0.01616273120518012252 ),
 .UNSPECIFIED. ) ;
#10601=CARTESIAN_POINT ( 'NONE',  ( 13.77203033081066685, -67.83931925369924443, -3.638954064322520665 ) ) ;
#10603=CARTESIAN_POINT ( 'NONE',  ( 12.36791015745245836, -52.24929059928631148, -3.199931146564426232 ) ) ;
#10611=ORIENTED_EDGE ( 'NONE', *, *, #987, .T. ) ;
#10614=EDGE_CURVE ( 'NONE', #8444, #11311, #4305, .T. ) ;
#10617=DIRECTION ( 'NONE',  ( 0.000000000000000000, 0.000000000000000000, 1.000000000000000000 ) ) ;
#10622=CARTESIAN_POINT ( 'NONE',  ( 19.97461805067967333, 0.000000000000000000, 4.000000000000001776 ) ) ;
#10631=AXIS2_PLACEMENT_3D ( 'NONE', #9897, #425, #14507 ) ;
#10634=AXIS2_PLACEMENT_3D ( 'NONE', #4276, #13600, #12373 ) ;
#10637=ORIENTED_EDGE ( 'NONE', *, *, #3576, .F. ) ;
#10645=EDGE_CURVE ( 'NONE', #5424, #2756, #4613, .T. ) ;
#10652=CARTESIAN_POINT ( 'NONE',  ( 32.72652119040196794, -55.34955111272466155, -2.958349455637756531 ) ) ;
#10657=CARTESIAN_POINT ( 'NONE',  ( 9.167948996869769829, -53.67524880067755078, -2.284438283807834758 ) ) ;
#10669=CARTESIAN_POINT ( 'NONE',  ( 32.60126426873069505, -53.72848551507535575, 3.102677277821895174 ) ) ;
#10671=ORIENTED_EDGE ( 'NONE', *, *, #6589, .T. ) ;
#10679=B_SPLINE_CURVE_WITH_KNOTS ( 'NONE', 3,
 ( #14734, #801, #9127, #5515, #5667, #13582, #3347, #8046, #13659, #10200, #13811, #12587, #6731, #3274, #12748, #6575, #7740, #643, #876, #7973, #3117, #2111, #6807 ),
 .UNSPECIFIED., .F., .F.,
 ( 4, 2, 2, 2, 2, 2, 2, 1, 2, 2, 2, 4 ),
 ( 0.000000000000000000, 0.0009744059347753146819, 0.001948811869550629364, 0.002436014836938296679, 0.002923217804325963995, 0.003897623739101298626, 0.004384826706488958135, 0.004872029673876616777, 0.005359232641264276287, 0.005846435608651934061, 0.006820841543427254815, 0.007795247478202574701 ),
 .UNSPECIFIED. ) ;
#10681=CARTESIAN_POINT ( 'NONE',  ( 9.351153736313083442, -54.69057383520976856, 3.126673503084359318 ) ) ;
#10691=CARTESIAN_POINT ( 'NONE',  ( 9.665751080312901422, -60.12777237996191104, -2.859594828286806667 ) ) ;
#10693=CARTESIAN_POINT ( 'NONE',  ( 27.79575038568464151, -66.12098470289355134, 4.407543342774871142 ) ) ;
#10717=CARTESIAN_POINT ( 'NONE',  ( 20.86173033120691045, -96.56299909827106376, 3.999999999999999112 ) ) ;
#10719=CARTESIAN_POINT ( 'NONE',  ( 27.69308748103538775, -66.48338622332397563, 4.442552071294104898 ) ) ;
#10721=CARTESIAN_POINT ( 'NONE',  ( 30.59224152647144024, -52.42016302384283222, -2.859972208321964970 ) ) ;
#10724=CIRCLE ( 'NONE', #15148, 6.000000000000000000 ) ;
#10726=ORIENTED_EDGE ( 'NONE', *, *, #9176, .F. ) ;
#10730=DIRECTION ( 'NONE',  ( -0.000000000000000000, -0.000000000000000000, -1.000000000000000000 ) ) ;
#10739=CARTESIAN_POINT ( 'NONE',  ( 31.72224702437784316, -52.94991738523431479, 2.538129127160420051 ) ) ;
#10745=CARTESIAN_POINT ( 'NONE',  ( 8.333746545461773181, -58.06117555224668081, 1.821720187977012628 ) ) ;
#10755=CARTESIAN_POINT ( 'NONE',  ( 8.766647633345350243, -57.08478275174014271, 2.747861298827293908 ) ) ;
#10756=AXIS2_PLACEMENT_3D ( 'NONE', #15092, #3546, #4541 ) ;
#10773=VERTEX_POINT ( 'NONE', #6781 ) ;
#10780=LINE ( 'NONE', #4928, #942 ) ;
#10782=FACE_OUTER_BOUND ( 'NONE', #8551, .T. ) ;
#10792=PLANE ( 'NONE',  #3381 ) ;
#10793=CARTESIAN_POINT ( 'NONE',  ( 24.10826840236108737, -69.39711819508849544, 6.201611931792130328 ) ) ;
#10796=CARTESIAN_POINT ( 'NONE',  ( 17.58146340911564920, -70.03159917004852275, 6.184016381206977719 ) ) ;
#10801=CARTESIAN_POINT ( 'NONE',  ( 33.42858924011148503, -55.21335607387715783, -1.971947758011750595 ) ) ;
#10803=AXIS2_PLACEMENT_3D ( 'NONE', #10262, #4403, #11178 ) ;
#10806=CARTESIAN_POINT ( 'NONE',  ( 32.48672609961973734, -59.22985212983979153, -2.757908476812882093 ) ) ;
#10807=ADVANCED_FACE ( 'NONE', ( #14182 ), #1166, .T. ) ;
#10808=SHAPE_REPRESENTATION_RELATIONSHIP ( 'NONE' , 'NONE' ,  #2630, #11812 ) ;
#10816=CARTESIAN_POINT ( 'NONE',  ( 33.10838500789091654, -54.46933172536108714, 2.097670533078143329 ) ) ;
#10829=CARTESIAN_POINT ( 'NONE',  ( 8.408558643351286221, -54.89597349494646750, 2.779010397565546242 ) ) ;
#10830=ADVANCED_FACE ( 'NONE', ( #7322 ), #10792, .F. ) ;
#10840=CARTESIAN_POINT ( 'NONE',  ( 11.45230383124209617, -61.78784708351296473, 3.496562482608114308 ) ) ;
#10841=EDGE_LOOP ( 'NONE', ( #7476, #8378, #15004, #14690 ) ) ;
#10845=ORIENTED_EDGE ( 'NONE', *, *, #1194, .T. ) ;
#10849=ADVANCED_FACE ( 'NONE', ( #7172 ), #14710, .T. ) ;
#10852=CIRCLE ( 'NONE', #4190, 2.000000000000000000 ) ;
#10856=CARTESIAN_POINT ( 'NONE',  ( 32.52281604437752804, -59.06479067038043240, 2.757123406423070744 ) ) ;
#10863=ORIENTED_EDGE ( 'NONE', *, *, #9501, .F. ) ;
#10865=DIRECTION ( 'NONE',  ( -1.000000000000000000, 0.000000000000000000, 0.000000000000000000 ) ) ;
#10872=ORIENTED_EDGE ( 'NONE', *, *, #10645, .F. ) ;
#10873=CARTESIAN_POINT ( 'NONE',  ( 6.633218499801108337, -47.02718879221286841, 2.731995254387804106 ) ) ;
#10880=CARTESIAN_POINT ( 'NONE',  ( 32.81365369610337979, -55.58532807872790471, -2.910983838681297620 ) ) ;
#10886=CARTESIAN_POINT ( 'NONE',  ( 32.54790116764300478, -57.26105658658105568, -1.816685854991389348 ) ) ;
#10904=CARTESIAN_POINT ( 'NONE',  ( 16.53849081582479741, -69.39711819508849544, -5.637959728397558656 ) ) ;
#10908=VERTEX_POINT ( 'NONE', #7621 ) ;
#10910=( BOUNDED_SURFACE ( )  B_SPLINE_SURFACE ( 3, 2, ( 
 ( #2995, #11148, #7687 ),
 ( #11213, #668, #10071 ),
 ( #14752, #4208, #2297 ),
 ( #13991, #9301, #9225 ),
 ( #972, #4439, #5533 ),
 ( #8067, #1059, #6989 ),
 ( #2135, #13758, #12767 ),
 ( #5686, #11679, #2214 ),
 ( #10218, #3139, #6674 ),
 ( #5453, #13838, #4524 ),
 ( #10377, #13909, #3448 ),
 ( #12610, #11360, #3213 ),
 ( #6828, #7918, #1974 ),
 ( #6906, #822, #2061 ),
 ( #12850, #9153, #897 ),
 ( #11514, #3370, #6748 ),
 ( #5772, #10147, #11598 ),
 ( #11433, #10453, #3294 ),
 ( #14835, #15144, #15076 ),
 ( #14905, #4599, #7838 ),
 ( #7989, #4281, #8982 ),
 ( #8142, #5609, #13680 ),
 ( #12531, #4366, #9064 ),
 ( #10301, #14992, #12683 ) ),
 .UNSPECIFIED., .F., .F., .F. ) 
 B_SPLINE_SURFACE_WITH_KNOTS ( ( 4, 2, 2, 2, 2, 2, 2, 2, 2, 2, 2, 4 ),
 ( 3, 3 ),
 ( 0.000000000000000000, 0.0007569831467696874674, 0.001513966293539374935, 0.002270949440309062185, 0.002649441013693906027, 0.003027932587078749870, 0.003406424160463593712, 0.003784915733848437120, 0.004541898880618124371, 0.004920390454002968213, 0.005298882027387812055, 0.006055865174157499739 ),
 ( 0.000000000000000000, 1.000000000000000000 ),
 .UNSPECIFIED. ) 
 GEOMETRIC_REPRESENTATION_ITEM ( )  RATIONAL_B_SPLINE_SURFACE ( (
 ( 1.000000000000000000, 0.6947298545087537969, 1.000000000000000000),
 ( 1.000000000000000000, 0.7030359819960353418, 1.000000000000000000),
 ( 1.000000000000000000, 0.7110141033721660841, 1.000000000000000000),
 ( 1.000000000000000000, 0.7265357204475634267, 1.000000000000000000),
 ( 1.000000000000000000, 0.7341632328269016572, 1.000000000000000000),
 ( 1.000000000000000000, 0.7486333683862642641, 1.000000000000000000),
 ( 1.000000000000000000, 0.7555062062384456656, 1.000000000000000000),
 ( 1.000000000000000000, 0.7654404118660548262, 1.000000000000000000),
 ( 1.000000000000000000, 0.7687038416332773183, 1.000000000000000000),
 ( 1.000000000000000000, 0.7749762558334875040, 1.000000000000000000),
 ( 1.000000000000000000, 0.7780012814122965192, 1.000000000000000000),
 ( 1.000000000000000000, 0.7838538191795068055, 1.000000000000000000),
 ( 1.000000000000000000, 0.7866813202764467716, 1.000000000000000000),
 ( 1.000000000000000000, 0.7921509987295783928, 1.000000000000000000),
 ( 1.000000000000000000, 0.7948100380743099436, 1.000000000000000000),
 ( 1.000000000000000000, 0.8023666703952255785, 1.000000000000000000),
 ( 1.000000000000000000, 0.8068432255864165237, 1.000000000000000000),
 ( 1.000000000000000000, 0.8126963150101534916, 1.000000000000000000),
 ( 1.000000000000000000, 0.8145123882374375457, 1.000000000000000000),
 ( 1.000000000000000000, 0.8177588193891082158, 1.000000000000000000),
 ( 1.000000000000000000, 0.8191832667250865674, 1.000000000000000000),
 ( 1.000000000000000000, 0.8228396104941049227, 1.000000000000000000),
 ( 1.000000000000000000, 0.8244610879124181224, 1.000000000000000000),
 ( 1.000000000000000000, 0.8250833044923663318, 1.000000000000000000) ) ) 
 REPRESENTATION_ITEM ( '' )  SURFACE ( )  );
#10914=CARTESIAN_POINT ( 'NONE',  ( 8.294871422301858033, -55.21335607387847944, 1.971947758013492535 ) ) ;
#10922=ORIENTED_EDGE ( 'NONE', *, *, #1858, .T. ) ;
#10927=EDGE_CURVE ( 'NONE', #2517, #15191, #6389, .T. ) ;
#10942=VERTEX_POINT ( 'NONE', #3007 ) ;
#10951=CARTESIAN_POINT ( 'NONE',  ( 13.13019313627999729, -57.14688517088755759, 4.208364643998075749 ) ) ;
#10953=CARTESIAN_POINT ( 'NONE',  ( 30.90276055061299232, -52.52652714576225890, 2.773109545209086590 ) ) ;
#10954=CARTESIAN_POINT ( 'NONE',  ( 31.72083858694995584, -52.95955415863809179, -2.537984986062459036 ) ) ;
#10957=DIRECTION ( 'NONE',  ( 0.000000000000000000, -1.000000000000000000, 0.000000000000000000 ) ) ;
#10958=CARTESIAN_POINT ( 'NONE',  ( 33.12582565096496268, -59.20619211347771937, -2.502190571104468741 ) ) ;
#10961=CARTESIAN_POINT ( 'NONE',  ( 9.348584929445154401, -54.69456399997502416, 3.125517714509065570 ) ) ;
#10968=CARTESIAN_POINT ( 'NONE',  ( 29.07175354616249052, -50.97709764759155604, -4.214141842619275380 ) ) ;
#10979=ORIENTED_EDGE ( 'NONE', *, *, #11318, .T. ) ;
#10986=DIRECTION ( 'NONE',  ( 0.000000000000000000, 0.000000000000000000, 1.000000000000000000 ) ) ;
#10988=( BOUNDED_SURFACE ( )  B_SPLINE_SURFACE ( 3, 2, ( 
 ( #13390, #5095, #10873 ),
 ( #2565, #14484, #9576 ),
 ( #2710, #1560, #13109 ),
 ( #1481, #7405, #2787 ),
 ( #7482, #8700, #4002 ),
 ( #8493, #10951, #6260 ),
 ( #11939, #3931, #2632 ),
 ( #9800, #9872, #2848 ),
 ( #8627, #12168, #7550 ),
 ( #10796, #8416, #1400 ),
 ( #12247, #176, #6108 ),
 ( #1627, #6327, #14554 ),
 ( #6187, #330, #256 ),
 ( #5024, #11020, #470 ) ),
 .UNSPECIFIED., .F., .F., .F. ) 
 B_SPLINE_SURFACE_WITH_KNOTS ( ( 4, 2, 2, 2, 2, 2, 4 ),
 ( 3, 3 ),
 ( 0.2948322565876035362, 0.2981287057529112827, 0.3014251549182189738, 0.3080180532488344669, 0.3146109515794499600, 0.3179074007447577066, 0.3212038499100654532 ),
 ( 0.000000000000000000, 0.9256633218932661666 ),
 .UNSPECIFIED. ) 
 GEOMETRIC_REPRESENTATION_ITEM ( )  RATIONAL_B_SPLINE_SURFACE ( (
 ( 1.000000000000000000, 0.9979219307738474987, 0.9996910464737041035),
 ( 1.000000000000000000, 0.9979571442240684487, 0.9996962817755321584),
 ( 1.000000000000000000, 0.9979896195972217665, 0.9997011099982531235),
 ( 1.000000000000000000, 0.9980478678147421956, 0.9997097699562453865),
 ( 1.000000000000000000, 0.9980736641738821024, 0.9997136051875368246),
 ( 1.000000000000000000, 0.9981411222205919254, 0.9997236344017447207),
 ( 1.000000000000000000, 0.9981728461536270025, 0.9997283509053414008),
 ( 1.000000000000000000, 0.9982102196781720282, 0.9997339073526689823),
 ( 1.000000000000000000, 0.9982158677593769847, 0.9997347470718578322),
 ( 1.000000000000000000, 0.9982052731646247068, 0.9997331719378983461),
 ( 1.000000000000000000, 0.9981985596398339489, 0.9997321738156357274),
 ( 1.000000000000000000, 0.9981789131846819929, 0.9997292529112105086),
 ( 1.000000000000000000, 0.9981660722458850499, 0.9997273438057426853),
 ( 1.000000000000000000, 0.9981504490785557682, 0.9997250210570212126) ) ) 
 REPRESENTATION_ITEM ( '' )  SURFACE ( )  );
#10990=ORIENTED_EDGE ( 'NONE', *, *, #5480, .F. ) ;
#10991=CARTESIAN_POINT ( 'NONE',  ( 28.75670713205263596, -65.20845675887582615, 3.989712384468892203 ) ) ;
#10993=ORIENTED_EDGE ( 'NONE', *, *, #14483, .F. ) ;
#10998=CARTESIAN_POINT ( 'NONE',  ( 27.67989258697571131, -66.53205946168593243, -4.446982897616444497 ) ) ;
#11000=ORIENTED_EDGE ( 'NONE', *, *, #12750, .T. ) ;
#11006=ORIENTED_EDGE ( 'NONE', *, *, #6088, .T. ) ;
#11013=CARTESIAN_POINT ( 'NONE',  ( 33.12442989620986822, -59.21224831720011395, -1.832439066039627251 ) ) ;
#11017=CARTESIAN_POINT ( 'NONE',  ( 13.86173033120691223, -69.39711819508849544, 2.500000000000000000 ) ) ;
#11018=AXIS2_PLACEMENT_3D ( 'NONE', #4855, #13166, #6173 ) ;
#11019=FACE_OUTER_BOUND ( 'NONE', #3282, .T. ) ;
#11020=CARTESIAN_POINT ( 'NONE',  ( 13.88313415068312118, -68.65142943889351557, 4.053691724355805270 ) ) ;
#11029=CARTESIAN_POINT ( 'NONE',  ( 32.64893181228500652, -58.48798588983608226, -2.754379989675052265 ) ) ;
#11048=DIRECTION ( 'NONE',  ( -0.000000000000000000, 1.000000000000000000, -0.000000000000000000 ) ) ;
#11057=CARTESIAN_POINT ( 'NONE',  ( 28.31271169503452256, -66.37912134690742505, 3.509717431438163171 ) ) ;
#11058=ORIENTED_EDGE ( 'NONE', *, *, #12234, .T. ) ;
#11063=FACE_OUTER_BOUND ( 'NONE', #6295, .T. ) ;
#11080=PLANE ( 'NONE',  #4812 ) ;
#11086=CARTESIAN_POINT ( 'NONE',  ( 13.15370223272280370, -65.65107448351760411, -3.408697305255636412 ) ) ;
#11095=CARTESIAN_POINT ( 'NONE',  ( 33.52235686305655804, -57.48563641131178770, -1.816685854991397564 ) ) ;
#11096=DIRECTION ( 'NONE',  ( 1.000000000000000000, 0.000000000000000000, 0.000000000000000000 ) ) ;
#11100=ADVANCED_FACE ( 'NONE', ( #10083 ), #4009, .T. ) ;
#11112=STYLED_ITEM('',(#15272),#14540);
#11124=CARTESIAN_POINT ( 'NONE',  ( 9.664729663202141552, -53.19870790407432537, 3.318692829847595505 ) ) ;
#11135=B_SPLINE_CURVE_WITH_KNOTS ( 'NONE', 3,
 ( #11762, #2377, #10840, #10540, #11911, #1371, #6075, #12857, #301, #9703, #7076, #3457, #12209, #12285 ),
 .UNSPECIFIED., .F., .F.,
 ( 4, 2, 2, 2, 2, 2, 4 ),
 ( 1.788112030672749005E-18, 0.002516897397286753553, 0.003775346095930122957, 0.005033794794573492361, 0.006292243493216862632, 0.007550692191860232903, 0.01006758958914701074 ),
 .UNSPECIFIED. ) ;
#11148=CARTESIAN_POINT ( 'NONE',  ( 12.02094163398139237, -52.24929059928630437, -4.175384597093462880 ) ) ;
#11151=EDGE_LOOP ( 'NONE', ( #3396, #2131, #24, #12737 ) ) ;
#11158=CARTESIAN_POINT ( 'NONE',  ( 13.86173033120691223, -69.39711819508849544, 2.500000000000000000 ) ) ;
#11171=DIRECTION ( 'NONE',  ( 0.000000000000000000, 0.000000000000000000, -1.000000000000000000 ) ) ;
#11172=CARTESIAN_POINT ( 'NONE',  ( 8.127555659019208179, -57.16650977415540069, -1.814547216390245632 ) ) ;
#11175=CARTESIAN_POINT ( 'NONE',  ( 17.09549820959326638, -82.24929059928629727, 1.347403282660979640 ) ) ;
#11178=DIRECTION ( 'NONE',  ( 0.000000000000000000, 0.000000000000000000, -1.000000000000000000 ) ) ;
#11181=CARTESIAN_POINT ( 'NONE',  ( 23.59140218557817192, -57.03285117764829693, -6.445925775548339232 ) ) ;
#11191=CARTESIAN_POINT ( 'NONE',  ( 12.92924986285039957, -63.81378734511389439, 4.043274055231490749 ) ) ;
#11199=DIRECTION ( 'NONE',  ( 0.000000000000000000, -1.000000000000000000, 0.000000000000000000 ) ) ;
#11202=EDGE_LOOP ( 'NONE', ( #2508, #13192, #4011, #666 ) ) ;
#11212=AXIS2_PLACEMENT_3D ( 'NONE', #10597, #13287, #3812 ) ;
#11213=CARTESIAN_POINT ( 'NONE',  ( 11.79320013990377802, -53.28555914635324342, -4.056187502120401689 ) ) ;
#11214=LINE ( 'NONE', #2062, #332 ) ;
#11223=( NAMED_UNIT ( * ) PLANE_ANGLE_UNIT ( ) SI_UNIT ( $, .RADIAN. ) );
#11236=FACE_OUTER_BOUND ( 'NONE', #14238, .T. ) ;
#11243=CARTESIAN_POINT ( 'NONE',  ( 28.24952126317575818, -64.89111109908230901, -4.244693487287873879 ) ) ;
#11248=CARTESIAN_POINT ( 'NONE',  ( 9.657759076947806776, -54.31552982368702942, 3.256647958671365917 ) ) ;
#11257=DIRECTION ( 'NONE',  ( -1.000000000000000000, 0.000000000000000000, 0.000000000000000000 ) ) ;
#11260=CARTESIAN_POINT ( 'NONE',  ( 13.86173033120691223, -69.39711819508849544, -3.619682905202625811 ) ) ;
#11268=DIRECTION ( 'NONE',  ( 0.000000000000000000, 1.000000000000000000, 0.000000000000000000 ) ) ;
#11273=CARTESIAN_POINT ( 'NONE',  ( 27.86203511185233594, -69.48056866272028742, 4.214447830835810649 ) ) ;
#11280=CARTESIAN_POINT ( 'NONE',  ( 27.86188286885952081, -69.45278782524461292, -3.616934341765170036 ) ) ;
#11282=B_SPLINE_CURVE_WITH_KNOTS ( 'NONE', 3,
 ( #3331, #11478, #10338, #7107 ),
 .UNSPECIFIED., .F., .F.,
 ( 4, 4 ),
 ( 0.000000000000000000, 0.001771361151111836311 ),
 .UNSPECIFIED. ) ;
#11286=CARTESIAN_POINT ( 'NONE',  ( 12.44985739169131556, -58.32476007869853873, 2.500000000000000000 ) ) ;
#11289=EDGE_CURVE ( 'NONE', #10251, #12406, #11990, .T. ) ;
#11290=ORIENTED_EDGE ( 'NONE', *, *, #14094, .F. ) ;
#11306=CARTESIAN_POINT ( 'NONE',  ( 20.86173033120691045, -72.24929059928631148, 0.000000000000000000 ) ) ;
#11307=CARTESIAN_POINT ( 'NONE',  ( 11.46205536272672454, -61.79747627231519402, -3.500139319476019750 ) ) ;
#11311=VERTEX_POINT ( 'NONE', #14528 ) ;
#11318=EDGE_CURVE ( 'NONE', #7093, #1111, #3978, .T. ) ;
#11319=CYLINDRICAL_SURFACE ( 'NONE', #2691, 7.000000000000000000 ) ;
#11320=EDGE_CURVE ( 'NONE', #11520, #2756, #14464, .T. ) ;
#11328=DIRECTION ( 'NONE',  ( 0.000000000000000000, 0.000000000000000000, 1.000000000000000000 ) ) ;
#11337=CARTESIAN_POINT ( 'NONE',  ( 12.61580082134570269, -64.50532980541186134, 3.862852061923984337 ) ) ;
#11341=CARTESIAN_POINT ( 'NONE',  ( 32.31055461597316025, -59.69871785856275181, 2.790504257380250319 ) ) ;
#11345=FACE_OUTER_BOUND ( 'NONE', #378, .T. ) ;
#11347=CARTESIAN_POINT ( 'NONE',  ( 17.40655560129473756, -73.00063092935795339, -6.088059227058379541 ) ) ;
#11351=CARTESIAN_POINT ( 'NONE',  ( 28.21768499689855503, -66.70046270226332297, 4.174231074483972570 ) ) ;
#11355=DIRECTION ( 'NONE',  ( 0.000000000000000000, -1.000000000000000000, 0.000000000000000000 ) ) ;
#11360=CARTESIAN_POINT ( 'NONE',  ( 8.844813971085542903, -54.08909618700739230, -2.984935890591794205 ) ) ;
#11365=ORIENTED_EDGE ( 'NONE', *, *, #9818, .T. ) ;
#11372=CIRCLE ( 'NONE', #9907, 31.00000000000000000 ) ;
#11380=LINE ( 'NONE', #14569, #2003 ) ;
#11381=ORIENTED_EDGE ( 'NONE', *, *, #11664, .F. ) ;
#11383=FACE_OUTER_BOUND ( 'NONE', #4073, .T. ) ;
#11385=CARTESIAN_POINT ( 'NONE',  ( 32.10796813252333948, -61.48517313025205766, 2.719255632294420799 ) ) ;
#11399=CARTESIAN_POINT ( 'NONE',  ( 32.94077818407075853, -56.07092277360308685, 2.830630916608660286 ) ) ;
#11404=CARTESIAN_POINT ( 'NONE',  ( 32.52281604437752804, -59.06479067038042530, 2.757123406423263923 ) ) ;
#11425=CYLINDRICAL_SURFACE ( 'NONE', #8751, 4.276034690655513337 ) ;
#11429=CARTESIAN_POINT ( 'NONE',  ( 27.85548922659567239, -68.67521603616586390, -4.260811380315422170 ) ) ;
#11433=CARTESIAN_POINT ( 'NONE',  ( 8.812572261450901223, -55.94973218888541311, -2.850075077558482661 ) ) ;
#11444=CARTESIAN_POINT ( 'NONE',  ( 9.200644618036294631, -59.06479067038042530, -2.757123406423266587 ) ) ;
#11445=DIRECTION ( 'NONE',  ( 0.000000000000000000, -0.000000000000000000, 1.000000000000000000 ) ) ;
#11448=CARTESIAN_POINT ( 'NONE',  ( 10.42235396810873027, -53.71233130651032894, -3.555899869131464719 ) ) ;
#11455=AXIS2_PLACEMENT_3D ( 'NONE', #12793, #6851, #5634 ) ;
#11456=DIRECTION ( 'NONE',  ( 0.7546336727145961376, -0.5961293309129300777, 0.2741493039031510648 ) ) ;
#11457=CARTESIAN_POINT ( 'NONE',  ( 31.67019424172517716, -63.64653881684405690, 2.711348815098903575 ) ) ;
#11465=LINE ( 'NONE', #5637, #8417 ) ;
#11477=CARTESIAN_POINT ( 'NONE',  ( 13.86173033120691045, -68.61243380581730378, 3.657093847832754818 ) ) ;
#11478=CARTESIAN_POINT ( 'NONE',  ( 8.948125790170779581, -57.91121052158847249, 2.751677492798614288 ) ) ;
#11480=AXIS2_PLACEMENT_3D ( 'NONE', #4582, #4506, #9283 ) ;
#11482=CARTESIAN_POINT ( 'NONE',  ( 32.87342042526285013, -60.00774340954441044, 2.531751357929999280 ) ) ;
#11483=CIRCLE ( 'NONE', #6339, 3.000000000000000888 ) ;
#11486=CARTESIAN_POINT ( 'NONE',  ( 23.10474973039555380, -52.24929059928630437, 5.564967562786275579 ) ) ;
#11492=DIRECTION ( 'NONE',  ( -0.000000000000000000, -1.000000000000000000, -0.000000000000000000 ) ) ;
#11498=CARTESIAN_POINT ( 'NONE',  ( 20.86173033120691045, -69.39711819508849544, 0.000000000000000000 ) ) ;
#11501=ORIENTED_EDGE ( 'NONE', *, *, #7909, .T. ) ;
#11503=ORIENTED_EDGE ( 'NONE', *, *, #2985, .T. ) ;
#11511=CARTESIAN_POINT ( 'NONE',  ( 27.32034923811608707, -68.64054039872385715, -4.542265185079617851 ) ) ;
#11512=ORIENTED_EDGE ( 'NONE', *, *, #1131, .T. ) ;
#11514=CARTESIAN_POINT ( 'NONE',  ( 8.990114402468742938, -55.34773484034933944, -2.956285999963581101 ) ) ;
#11520=VERTEX_POINT ( 'NONE', #10062 ) ;
#11536=CARTESIAN_POINT ( 'NONE',  ( 24.14199725329817880, -70.03159917007936031, 6.184016381206977719 ) ) ;
#11540=CARTESIAN_POINT ( 'NONE',  ( 18.24487436548682595, -52.24929059928630437, 6.492462156583967747 ) ) ;
#11556=B_SPLINE_CURVE_WITH_KNOTS ( 'NONE', 3,
 ( #5041, #5334, #1646, #6345, #14501, #5183, #627, #414 ),
 .UNSPECIFIED., .F., .F.,
 ( 4, 2, 2, 4 ),
 ( 0.000000000000000000, 0.0002685268308981138730, 0.0005370536617962277460, 0.001074107323592453107 ),
 .UNSPECIFIED. ) ;
#11560=CARTESIAN_POINT ( 'NONE',  ( 31.49298359385885959, -60.71197230342421136, 3.050751728647424610 ) ) ;
#11577=LINE ( 'NONE', #10127, #14037 ) ;
#11578=B_SPLINE_CURVE_WITH_KNOTS ( 'NONE', 3,
 ( #9976, #6429, #13661, #7664 ),
 .UNSPECIFIED., .F., .F.,
 ( 4, 4 ),
 ( 0.0005996816226311996569, 0.004245596575621808817 ),
 .UNSPECIFIED. ) ;
#11580=DIRECTION ( 'NONE',  ( -0.3351302520855081735, 0.000000000000000000, 0.9421718071228324387 ) ) ;
#11582=CARTESIAN_POINT ( 'NONE',  ( 10.05326642068865262, -63.64653881684382952, -2.711348815098831633 ) ) ;
#11598=CARTESIAN_POINT ( 'NONE',  ( 8.286281640854550545, -55.20947656326016073, -1.969991847666946905 ) ) ;
#11618=ORIENTED_EDGE ( 'NONE', *, *, #2739, .F. ) ;
#11621=CARTESIAN_POINT ( 'NONE',  ( 18.24487436548682950, -53.24929059928630437, -6.492462156583989064 ) ) ;
#11622=CARTESIAN_POINT ( 'NONE',  ( 28.85634326780420267, -53.69151354803189946, 4.215873133687699337 ) ) ;
#11634=CARTESIAN_POINT ( 'NONE',  ( 30.60592481596644632, -62.41236107492795782, 2.580051240451675554 ) ) ;
#11635=ORIENTED_EDGE ( 'NONE', *, *, #5264, .T. ) ;
#11643=CARTESIAN_POINT ( 'NONE',  ( 23.69232253801246557, -82.24929059928629727, -4.472107801411126182 ) ) ;
#11648=CARTESIAN_POINT ( 'NONE',  ( 10.49322424505076690, -52.67209071833767808, -2.680141711508894353 ) ) ;
#11649=CARTESIAN_POINT ( 'NONE',  ( 10.49550990701181696, -52.67117483538238787, 2.680786716676139214 ) ) ;
#11656=CARTESIAN_POINT ( 'NONE',  ( 20.86173033120691045, -69.39711819508849544, 0.000000000000000000 ) ) ;
#11658=CARTESIAN_POINT ( 'NONE',  ( 9.286411473068065803, -59.38916093354925607, 2.764669745501079579 ) ) ;
#11659=CARTESIAN_POINT ( 'NONE',  ( 30.85913393947397054, -53.50034303113434930, 3.720434809418716515 ) ) ;
#11661=EDGE_LOOP ( 'NONE', ( #14916, #314, #1799, #8515 ) ) ;
#11664=EDGE_CURVE ( 'NONE', #13577, #13900, #2864, .T. ) ;
#11669=CARTESIAN_POINT ( 'NONE',  ( 14.30639712155258003, -67.71210253279622293, -4.528315385689293926 ) ) ;
#11675=ORIENTED_EDGE ( 'NONE', *, *, #10082, .F. ) ;
#11679=CARTESIAN_POINT ( 'NONE',  ( 9.438813863662174342, -53.39687877504488966, -3.230473295589093130 ) ) ;
#11697=CARTESIAN_POINT ( 'NONE',  ( 23.53111059738935040, -55.08889408822823697, 6.471126372660433113 ) ) ;
#11700=EDGE_CURVE ( 'NONE', #8652, #5446, #7045, .T. ) ;
#11709=CARTESIAN_POINT ( 'NONE',  ( 28.56964104117922076, -65.59433601606471598, 3.409308316089453506 ) ) ;
#11710=ORIENTED_EDGE ( 'NONE', *, *, #3896, .F. ) ;
#11719=EDGE_CURVE ( 'NONE', #1828, #302, #82, .T. ) ;
#11724=CARTESIAN_POINT ( 'NONE',  ( 8.989437364795538343, -53.88923483553375604, -2.226753743598178570 ) ) ;
#11730=B_SPLINE_CURVE_WITH_KNOTS ( 'NONE', 3,
 ( #13955, #2251, #10184, #12891, #6951, #4640, #1092, #5803 ),
 .UNSPECIFIED., .F., .F.,
 ( 4, 2, 2, 4 ),
 ( 1.788112030672749005E-18, 0.0006709104321108792356, 0.001341820864221756737, 0.002683641728443497427 ),
 .UNSPECIFIED. ) ;
#11736=AXIS2_PLACEMENT_3D ( 'NONE', #9763, #13291, #5205 ) ;
#11738=CARTESIAN_POINT ( 'NONE',  ( 9.665531796221262795, -60.12744825561600948, 2.859530283892859348 ) ) ;
#11740=CARTESIAN_POINT ( 'NONE',  ( 32.73334625994522185, -55.34773484034921864, 2.956285999963537581 ) ) ;
#11741=VERTEX_POINT ( 'NONE', #11175 ) ;
#11747=ORIENTED_EDGE ( 'NONE', *, *, #14094, .T. ) ;
#11749=CARTESIAN_POINT ( 'NONE',  ( 20.86173033120691045, -85.24929059928631148, 0.000000000000000000 ) ) ;
#11751=CARTESIAN_POINT ( 'NONE',  ( 14.09856246968317528, -52.24929059928631148, -4.899481419395764981 ) ) ;
#11760=CARTESIAN_POINT ( 'NONE',  ( 32.77533165178194707, -57.91122518709860856, 2.751677560523507982 ) ) ;
#11762=CARTESIAN_POINT ( 'NONE',  ( 10.23047706855496841, -60.71197230342421136, 3.050751728647412175 ) ) ;
#11778=DIRECTION ( 'NONE',  ( -0.3351302520855081735, 0.000000000000000000, -0.9421718071228324387 ) ) ;
#11789=B_SPLINE_CURVE_WITH_KNOTS ( 'NONE', 3,
 ( #8116, #14962, #6799, #1025, #1945, #13648, #9270, #12816, #3267, #13965, #9200, #2262, #11649, #945, #5419, #12739, #5657, #5506 ),
 .UNSPECIFIED., .F., .F.,
 ( 4, 2, 2, 2, 2, 2, 2, 2, 4 ),
 ( 0.0009656645577509051157, 0.001819362422807364790, 0.002673060287863824463, 0.003526758152920284571, 0.004380456017976744679, 0.005234153883033203919, 0.006087851748089664027, 0.006941549613146123267, 0.007795247478202583374 ),
 .UNSPECIFIED. ) ;
#11792=CARTESIAN_POINT ( 'NONE',  ( 29.49572703012646357, -62.74876579108524766, 3.782929430830329842 ) ) ;
#11795=CARTESIAN_POINT ( 'NONE',  ( 31.31200846133606319, -52.71989690418642027, -2.656489712860274466 ) ) ;
#11800=CARTESIAN_POINT ( 'NONE',  ( 18.08359295236611786, -58.63441909321034728, 6.426091441073436883 ) ) ;
#11802=DIRECTION ( 'NONE',  ( 0.2245716668862459686, -0.9744202983869693080, 0.008523410314123252077 ) ) ;
#11807=DIRECTION ( 'NONE',  ( -1.000000000000000000, -0.000000000000000000, -0.000000000000000000 ) ) ;
#11810=CARTESIAN_POINT ( 'NONE',  ( 33.47477952685317604, -55.33002571195186903, 2.691408569078770796 ) ) ;
#11812=ADVANCED_BREP_SHAPE_REPRESENTATION ( '', ( #14540, #6315 ), #5577 ) ;
#11819=CARTESIAN_POINT ( 'NONE',  ( 19.97461805067967688, -82.24929059928629727, -4.000000000000000888 ) ) ;
#11825=CARTESIAN_POINT ( 'NONE',  ( 9.025688005465005048, -53.84505747417151156, 3.062469901903004388 ) ) ;
#11829=ORIENTED_EDGE ( 'NONE', *, *, #12773, .F. ) ;
#11833=ORIENTED_EDGE ( 'NONE', *, *, #11320, .F. ) ;
#11846=CARTESIAN_POINT ( 'NONE',  ( 29.35555050496136431, -52.24929059928631148, -3.199931146564432449 ) ) ;
#11849=EDGE_LOOP ( 'NONE', ( #7360, #2761, #8160, #11829, #10611, #1062, #14269, #6817 ) ) ;
#11857=AXIS2_PLACEMENT_3D ( 'NONE', #9103, #8944, #10101 ) ;
#11861=DIRECTION ( 'NONE',  ( 0.000000000000000000, 0.000000000000000000, 1.000000000000000000 ) ) ;
#11864=CARTESIAN_POINT ( 'NONE',  ( 8.948129010626443502, -57.91122518709997991, 2.751677560521355037 ) ) ;
#11865=CARTESIAN_POINT ( 'NONE',  ( 23.47858629692700916, -53.24929059928630437, -6.492462156583981070 ) ) ;
#11868=CARTESIAN_POINT ( 'NONE',  ( 33.02192861186179584, -59.65700314074641852, -1.835602613601381883 ) ) ;
#11872=AXIS2_PLACEMENT_3D ( 'NONE', #11306, #14776, #8703 ) ;
#11902=ORIENTED_EDGE ( 'NONE', *, *, #1913, .F. ) ;
#11911=CARTESIAN_POINT ( 'NONE',  ( 12.46522364980626918, -63.07964102605459544, 3.871020209143785529 ) ) ;
#11920=ORIENTED_EDGE ( 'NONE', *, *, #13970, .T. ) ;
#11932=CLOSED_SHELL ( 'NONE', ( #3897, #430, #14456, #7644, #5277, #10173, #3134, #309, #5154, #13247, #5723, #9318, #12705, #6985, #8000, #4915, #926, #7808, #9803, #12847, #2619, #7957, #8209, #843, #3584, #3545, #11100, #3814, #2689, #5678, #7849, #13940, #3492, #9314, #814, #12503, #8746, #8243, #7601, #7123, #6130, #448, #8659, #18, #10849, #7890, #4093, #13324, #1145, #10807, #3080, #1597, #12059, #10830, #9336, #7288, #4700, #1977, #9819, #6262, #5526, #4489 ) ) ;
#11939=CARTESIAN_POINT ( 'NONE',  ( 17.93383279432583421, -62.59345883551662126, 6.358786672824582098 ) ) ;
#11942=CARTESIAN_POINT ( 'NONE',  ( 31.47353884241217159, -52.79727339576417222, 2.610417277227879307 ) ) ;
#11944=CARTESIAN_POINT ( 'NONE',  ( 32.39362946278320976, -53.50309148220193833, -3.187126068577873728 ) ) ;
#11951=DIRECTION ( 'NONE',  ( 0.9744556954135530358, 0.2245798247307374262, 0.000000000000000000 ) ) ;
#11961=CARTESIAN_POINT ( 'NONE',  ( 31.94053544990188342, -53.09518070810378987, 3.364836540203623549 ) ) ;
#11968=VERTEX_POINT ( 'NONE', #4942 ) ;
#11978=CARTESIAN_POINT ( 'NONE',  ( 20.86173033120691045, -53.24929059928630437, 0.000000000000000000 ) ) ;
#11980=ORIENTED_EDGE ( 'NONE', *, *, #5937, .T. ) ;
#11986=VERTEX_POINT ( 'NONE', #10569 ) ;
#11990=LINE ( 'NONE', #2683, #5568 ) ;
#11991=CARTESIAN_POINT ( 'NONE',  ( 20.86173033120691045, -57.24929059928630437, 3.000000000000000888 ) ) ;
#11992=ORIENTED_EDGE ( 'NONE', *, *, #9039, .T. ) ;
#12002=AXIS2_PLACEMENT_3D ( 'NONE', #11656, #8123, #126 ) ;
#12004=FACE_OUTER_BOUND ( 'NONE', #829, .T. ) ;
#12009=SHAPE_DEFINITION_REPRESENTATION ( #2041, #2630 ) ;
#12010=DIRECTION ( 'NONE',  ( -1.000000000000000000, 0.000000000000000000, -0.000000000000000000 ) ) ;
#12016=CARTESIAN_POINT ( 'NONE',  ( 32.48858144966465744, -60.63355790302721715, 1.939046661991518095 ) ) ;
#12020=CARTESIAN_POINT ( 'NONE',  ( 32.05323433862615445, -54.31204422905957330, -3.261005077968392563 ) ) ;
#12026=CARTESIAN_POINT ( 'NONE',  ( 33.12442989620986822, -59.21224831720011395, 2.500000000000000000 ) ) ;
#12040=ORIENTED_EDGE ( 'NONE', *, *, #4744, .T. ) ;
#12044=CARTESIAN_POINT ( 'NONE',  ( 15.46081644285383483, -69.39711819508849544, -5.076148092048929250 ) ) ;
#12059=ADVANCED_FACE ( 'NONE', ( #11019 ), #11080, .F. ) ;
#12069=CARTESIAN_POINT ( 'NONE',  ( 14.09856246968322147, -52.24929059928629727, 4.899481419391097603 ) ) ;
#12073=DIRECTION ( 'NONE',  ( -1.000000000000000000, -0.000000000000000000, -0.000000000000000000 ) ) ;
#12076=CARTESIAN_POINT ( 'NONE',  ( 28.56975842969204038, -65.65107448351471930, -3.408697305255637300 ) ) ;
#12105=CARTESIAN_POINT ( 'NONE',  ( 32.21801100873970114, -53.34475964609211474, -2.389227176380471551 ) ) ;
#12112=CARTESIAN_POINT ( 'NONE',  ( 32.77533165179128360, -57.91122518710081124, -2.751677560519801169 ) ) ;
#12122=CARTESIAN_POINT ( 'NONE',  ( 33.74207955331441156, -53.52407281596779143, -2.732083154000400693 ) ) ;
#12127=DIRECTION ( 'NONE',  ( 0.000000000000000000, -1.000000000000000000, 0.000000000000000000 ) ) ;
#12129=ORIENTED_EDGE ( 'NONE', *, *, #10614, .T. ) ;
#12134=CARTESIAN_POINT ( 'NONE',  ( 9.047572573828887244, -55.23312247377393192, 2.984220967394216828 ) ) ;
#12137=CARTESIAN_POINT ( 'NONE',  ( 21.74884261173415467, -82.24929059928629727, -4.000000000000000888 ) ) ;
#12147=CARTESIAN_POINT ( 'NONE',  ( 25.53229935574759679, -53.25924492462442572, 5.664691252382116460 ) ) ;
#12153=EDGE_CURVE ( 'NONE', #11311, #3243, #8342, .T. ) ;
#12154=CARTESIAN_POINT ( 'NONE',  ( 27.79575038568401268, -66.12098470289947727, -4.407543342774902229 ) ) ;
#12159=VERTEX_POINT ( 'NONE', #6760 ) ;
#12167=DIRECTION ( 'NONE',  ( 0.000000000000000000, -0.000000000000000000, -1.000000000000000000 ) ) ;
#12168=CARTESIAN_POINT ( 'NONE',  ( 13.56565975558667247, -63.36830850588443553, 4.156137255536471287 ) ) ;
#12169=B_SPLINE_CURVE_WITH_KNOTS ( 'NONE', 3,
 ( #11846, #14239, #4776, #7085 ),
 .UNSPECIFIED., .F., .F.,
 ( 4, 4 ),
 ( 0.000000000000000000, 0.006683255761480911238 ),
 .UNSPECIFIED. ) ;
#12172=CARTESIAN_POINT ( 'NONE',  ( 33.63127143586577716, -56.35534736560776992, 1.852150208425979105 ) ) ;
#12173=CARTESIAN_POINT ( 'NONE',  ( 13.86797143582181491, -68.67521603617278458, -4.260811380361852585 ) ) ;
#12174=CARTESIAN_POINT ( 'NONE',  ( 27.33382790127958728, -69.39711819508849544, 4.502057496415716287 ) ) ;
#12180=CARTESIAN_POINT ( 'NONE',  ( 11.08747240253766897, -53.42215338339673281, 3.801984355195809240 ) ) ;
#12181=DIRECTION ( 'NONE',  ( 0.9421718071228325497, 2.933300018044979975E-16, 0.3351302520855077294 ) ) ;
#12184=CARTESIAN_POINT ( 'NONE',  ( 8.597635011448856446, -59.20619211347771937, -2.502190571104460748 ) ) ;
#12187=CARTESIAN_POINT ( 'NONE',  ( 29.14641708242553619, -50.05591495609735375, -4.211963358982893091 ) ) ;
#12209=CARTESIAN_POINT ( 'NONE',  ( 14.39660873059139767, -68.54636829475870741, 4.542647641079955001 ) ) ;
#12213=AXIS2_PLACEMENT_3D ( 'NONE', #12928, #2220, #15080 ) ;
#12219=CIRCLE ( 'NONE', #2875, 6.000000000000000000 ) ;
#12227=VECTOR ( 'NONE', #13365, 1000.000000000000000 ) ;
#12231=ORIENTED_EDGE ( 'NONE', *, *, #6143, .F. ) ;
#12233=ORIENTED_EDGE ( 'NONE', *, *, #7272, .T. ) ;
#12234=EDGE_CURVE ( 'NONE', #12856, #8652, #759, .T. ) ;
#12239=CARTESIAN_POINT ( 'NONE',  ( 19.97461805067967688, -82.24929059928629727, -6.000000000000000888 ) ) ;
#12245=CARTESIAN_POINT ( 'NONE',  ( 8.821484763567294607, -57.33450387999030795, -2.749014434309871469 ) ) ;
#12246=ORIENTED_EDGE ( 'NONE', *, *, #1236, .T. ) ;
#12247=CARTESIAN_POINT ( 'NONE',  ( 17.53865101127114201, -70.79589105106622071, 6.161139702144408758 ) ) ;
#12249=CARTESIAN_POINT ( 'NONE',  ( 33.07363029493502182, -59.43266865480772765, 1.834006918418328524 ) ) ;
#12255=CARTESIAN_POINT ( 'NONE',  ( 33.52366768382369600, -57.47994873761392398, -2.501453769636603486 ) ) ;
#12259=CARTESIAN_POINT ( 'NONE',  ( 8.741728328725566044, -56.83124152802056983, 2.758380730586871277 ) ) ;
#12264=CARTESIAN_POINT ( 'NONE',  ( 30.60592481596645342, -62.41236107492795782, -2.580051240451693317 ) ) ;
#12266=CARTESIAN_POINT ( 'NONE',  ( 24.01697609495870367, -67.68160391992793734, -6.249260988559870000 ) ) ;
#12272=ORIENTED_EDGE ( 'NONE', *, *, #5899, .F. ) ;
#12273=DIRECTION ( 'NONE',  ( -9.912705577010326536E-16, 0.000000000000000000, 1.000000000000000000 ) ) ;
#12276=AXIS2_PLACEMENT_3D ( 'NONE', #5497, #12646, #13956 ) ;
#12277=CARTESIAN_POINT ( 'NONE',  ( 11.84453356674751845, -63.30956378474061808, 2.875213255991846406 ) ) ;
#12278=CARTESIAN_POINT ( 'NONE',  ( 12.05519880765550411, -52.24929059928630437, 3.114712537286230098 ) ) ;
#12283=CARTESIAN_POINT ( 'NONE',  ( 9.276103490588601730, -60.71989949371947404, 2.646748467230720436 ) ) ;
#12285=CARTESIAN_POINT ( 'NONE',  ( 14.38963276113423895, -69.39711819508849544, 4.502057496415707405 ) ) ;
#12291=EDGE_CURVE ( 'NONE', #15191, #2378, #12169, .T. ) ;
#12297=CARTESIAN_POINT ( 'NONE',  ( 31.12893072307018016, -61.89517205449885751, -2.369674354392826920 ) ) ;
#12299=CARTESIAN_POINT ( 'NONE',  ( 23.10474973039555380, -52.24929059928630437, 5.564967562786275579 ) ) ;
#12303=ORIENTED_EDGE ( 'NONE', *, *, #13970, .F. ) ;
#12306=ORIENTED_EDGE ( 'NONE', *, *, #2754, .F. ) ;
#12307=VERTEX_POINT ( 'NONE', #3542 ) ;
#12331=CARTESIAN_POINT ( 'NONE',  ( 8.091875466796945915, -56.84639887601247921, -1.823510762986219058 ) ) ;
#12347=CARTESIAN_POINT ( 'NONE',  ( 29.69047892279256473, -53.28399145779480506, -4.141535524925036960 ) ) ;
#12353=VECTOR ( 'NONE', #4756, 1000.000000000000000 ) ;
#12355=CARTESIAN_POINT ( 'NONE',  ( 10.45251858057167915, -61.76394201828934882, 3.065891788195822976 ) ) ;
#12371=AXIS2_PLACEMENT_3D ( 'NONE', #11498, #3579, #5824 ) ;
#12373=DIRECTION ( 'NONE',  ( 0.000000000000000000, 0.000000000000000000, -1.000000000000000000 ) ) ;
#12377=DIRECTION ( 'NONE',  ( -1.000000000000000000, 0.000000000000000000, 0.000000000000000000 ) ) ;
#12388=B_SPLINE_CURVE_WITH_KNOTS ( 'NONE', 3,
 ( #8485, #13385, #6100, #7542, #2622, #6319, #7318, #11013 ),
 .UNSPECIFIED., .F., .F.,
 ( 4, 2, 2, 4 ),
 ( 8.673617379884035472E-19, 0.0006709104321108796693, 0.001341820864221758471, 0.002683641728443498728 ),
 .UNSPECIFIED. ) ;
#12390=FACE_BOUND ( 'NONE', #14696, .T. ) ;
#12398=CARTESIAN_POINT ( 'NONE',  ( 10.59452993935777165, -61.89517205451002013, -2.369674354332441446 ) ) ;
#12406=VERTEX_POINT ( 'NONE', #7305 ) ;
#12416=CARTESIAN_POINT ( 'NONE',  ( 27.62489819270789582, -52.24929059928629727, -4.899481419331793042 ) ) ;
#12423=CARTESIAN_POINT ( 'NONE',  ( 13.49335920019251134, -64.93526722763070325, 4.251815205945346676 ) ) ;
#12431=CARTESIAN_POINT ( 'NONE',  ( 9.976190356295422390, -60.51242536180875931, 2.958269724473149065 ) ) ;
#12433=CARTESIAN_POINT ( 'NONE',  ( 32.82061086202445921, -55.58404325705457438, -2.908775817946459785 ) ) ;
#12434=ORIENTED_EDGE ( 'NONE', *, *, #580, .T. ) ;
#12436=AXIS2_PLACEMENT_3D ( 'NONE', #1163, #10480, #9482 ) ;
#12455=AXIS2_PLACEMENT_3D ( 'NONE', #2647, #7418, #407 ) ;
#12458=CARTESIAN_POINT ( 'NONE',  ( 27.76589651684735927, -69.39711819508849544, 4.056575093033438328 ) ) ;
#12464=( BOUNDED_SURFACE ( )  B_SPLINE_SURFACE ( 3, 2, ( 
 ( #6296, #14306, #13153 ),
 ( #9547, #13298, #374 ),
 ( #3757, #14386, #1532 ),
 ( #6237, #3827, #13234 ),
 ( #8469, #2605, #2681 ),
 ( #5067, #13078, #14461 ),
 ( #14525, #3905, #8601 ),
 ( #2760, #10991, #447 ),
 ( #6010, #5140, #2456 ),
 ( #10693, #4837, #11057 ),
 ( #13436, #11351, #1964 ),
 ( #5524, #6662, #3058 ),
 ( #6440, #14596, #6511 ),
 ( #512, #11273, #10211 ) ),
 .UNSPECIFIED., .F., .F., .F. ) 
 B_SPLINE_SURFACE_WITH_KNOTS ( ( 4, 2, 2, 2, 2, 2, 4 ),
 ( 3, 3 ),
 ( 0.000000000000000000, 0.002560658414910374665, 0.003840987622365561998, 0.005121316829820749331, 0.006401646037275936230, 0.007681975244731123996, 0.01024263365964149866 ),
 ( 0.000000000000000000, 1.000000000000000000 ),
 .UNSPECIFIED. ) 
 GEOMETRIC_REPRESENTATION_ITEM ( )  RATIONAL_B_SPLINE_SURFACE ( (
 ( 1.000000000000000000, 0.8053615646146035090, 1.000000000000000000),
 ( 1.000000000000000000, 0.8105996499491424645, 1.000000000000000000),
 ( 1.000000000000000000, 0.8160199193853241439, 1.000000000000000000),
 ( 1.000000000000000000, 0.8240376314735337049, 1.000000000000000000),
 ( 1.000000000000000000, 0.8266971106454457097, 1.000000000000000000),
 ( 1.000000000000000000, 0.8319110421178486092, 1.000000000000000000),
 ( 1.000000000000000000, 0.8344214672177644454, 1.000000000000000000),
 ( 1.000000000000000000, 0.8392107060239341054, 1.000000000000000000),
 ( 1.000000000000000000, 0.8414897010531580124, 1.000000000000000000),
 ( 1.000000000000000000, 0.8457750297010538931, 1.000000000000000000),
 ( 1.000000000000000000, 0.8477871175333944187, 1.000000000000000000),
 ( 1.000000000000000000, 0.8533050377659684438, 1.000000000000000000),
 ( 1.000000000000000000, 0.8561733496717280900, 1.000000000000000000),
 ( 1.000000000000000000, 0.8581891718822901582, 1.000000000000000000) ) ) 
 REPRESENTATION_ITEM ( '' )  SURFACE ( )  );
#12470=CARTESIAN_POINT ( 'NONE',  ( 33.62917719264643068, -56.86702399164118304, -2.513921072345373542 ) ) ;
#12473=CARTESIAN_POINT ( 'NONE',  ( 13.13160920566000023, -64.18054652438912910, -4.118450070759328341 ) ) ;
#12475=AXIS2_PLACEMENT_3D ( 'NONE', #3402, #4241, #12562 ) ;
#12476=CARTESIAN_POINT ( 'NONE',  ( 32.97619012053721121, -56.45473609427280337, 2.788978005137584315 ) ) ;
#12486=CARTESIAN_POINT ( 'NONE',  ( 19.97461805067967333, -85.24929059928631148, 6.000000000000001776 ) ) ;
#12491=CARTESIAN_POINT ( 'NONE',  ( 29.93210037042245375, -53.28557117198399595, 4.055532625545659187 ) ) ;
#12495=CARTESIAN_POINT ( 'NONE',  ( 32.44676321640788075, -60.72048491829421124, 2.646952986714198097 ) ) ;
#12500=CARTESIAN_POINT ( 'NONE',  ( 20.86173033120691045, -53.24929059928630437, 7.000000000000000000 ) ) ;
#12502=CARTESIAN_POINT ( 'NONE',  ( 13.65275068252399571, -65.32322779889722142, 4.310009693575397982 ) ) ;
#12503=ADVANCED_FACE ( 'NONE', ( #11063 ), #8349, .T. ) ;
#12504=CARTESIAN_POINT ( 'NONE',  ( 10.83536516265427352, -52.51002131803453210, 3.753497227305226946 ) ) ;
#12505=CARTESIAN_POINT ( 'NONE',  ( 31.73919081233200856, -60.50127194134182673, 2.962969586007845102 ) ) ;
#12512=CARTESIAN_POINT ( 'NONE',  ( 17.78537369493905373, -66.03679020173537140, -6.288305159854754578 ) ) ;
#12516=CARTESIAN_POINT ( 'NONE',  ( 31.50598280721104416, -53.84004999663768132, -3.478067438360130215 ) ) ;
#12523=CARTESIAN_POINT ( 'NONE',  ( 12.36791015745245836, -52.24929059928631148, 2.500000000000000000 ) ) ;
#12524=EDGE_CURVE ( 'NONE', #8767, #8156, #10065, .T. ) ;
#12526=ORIENTED_EDGE ( 'NONE', *, *, #14267, .F. ) ;
#12531=CARTESIAN_POINT ( 'NONE',  ( 8.766501742169731770, -57.08411837894907848, -2.747858231244113991 ) ) ;
#12543=CARTESIAN_POINT ( 'NONE',  ( 9.974161267552085874, -60.51083307721924598, -2.957531760941039423 ) ) ;
#12544=CARTESIAN_POINT ( 'NONE',  ( 31.72322230991231962, -61.42570632716525125, 2.132522520905362651 ) ) ;
#12548=FACE_BOUND ( 'NONE', #7979, .T. ) ;
#12552=CARTESIAN_POINT ( 'NONE',  ( 31.88039071915910583, -62.60658208069056485, 2.715520055361023477 ) ) ;
#12553=ORIENTED_EDGE ( 'NONE', *, *, #4142, .F. ) ;
#12558=( BOUNDED_SURFACE ( )  B_SPLINE_SURFACE ( 3, 2, ( 
 ( #5907, #3804, #9677 ),
 ( #14364, #7199, #12983 ),
 ( #7273, #2658, #14281 ),
 ( #4745, #3731, #129 ),
 ( #11659, #8443, #6053 ),
 ( #9360, #12908, #4968 ),
 ( #10517, #11961, #10739 ),
 ( #15206, #9442, #4815 ),
 ( #276, #4662, #14133 ),
 ( #14053, #10669, #9515 ),
 ( #1201, #201, #13129 ),
 ( #8214, #2432, #1424 ),
 ( #6129, #2583, #8286 ),
 ( #13053, #3580, #2351 ),
 ( #14210, #7043, #10816 ),
 ( #11740, #10589, #7127 ),
 ( #3663, #11810, #1270 ),
 ( #5984, #4892, #5482 ),
 ( #6479, #13551, #1780 ),
 ( #7864, #6699, #4157 ),
 ( #12476, #10094, #3019 ),
 ( #7712, #617, #5322 ),
 ( #9951, #14938, #6210 ),
 ( #768, #4393, #10020 ) ),
 .UNSPECIFIED., .F., .F., .F. ) 
 B_SPLINE_SURFACE_WITH_KNOTS ( ( 4, 2, 2, 2, 2, 2, 2, 2, 2, 2, 2, 4 ),
 ( 3, 3 ),
 ( 0.000000000000000000, 0.0007569831467696884432, 0.001513966293539376886, 0.002270949440309065221, 0.002649441013693909497, 0.003027932587078753773, 0.003406424160463598048, 0.003784915733848441891, 0.004541898880618130442, 0.004920390454002974284, 0.005298882027387818994, 0.006055865174157507545 ),
 ( 0.000000000000000000, 1.000000000000000000 ),
 .UNSPECIFIED. ) 
 GEOMETRIC_REPRESENTATION_ITEM ( )  RATIONAL_B_SPLINE_SURFACE ( (
 ( 1.000000000000000000, 0.6947298545087511323, 1.000000000000000000),
 ( 1.000000000000000000, 0.7030359819960161349, 1.000000000000000000),
 ( 1.000000000000000000, 0.7110141033721932846, 1.000000000000000000),
 ( 1.000000000000000000, 0.7265357204475346720, 1.000000000000000000),
 ( 1.000000000000000000, 0.7341632328267053698, 1.000000000000000000),
 ( 1.000000000000000000, 0.7486333683864616617, 1.000000000000000000),
 ( 1.000000000000000000, 0.7555062062380646370, 1.000000000000000000),
 ( 1.000000000000000000, 0.7654404118662447853, 1.000000000000000000),
 ( 1.000000000000000000, 0.7687038416331641866, 1.000000000000000000),
 ( 1.000000000000000000, 0.7749762558335999696, 1.000000000000000000),
 ( 1.000000000000000000, 0.7780012814123101750, 1.000000000000000000),
 ( 1.000000000000000000, 0.7838538191794924836, 1.000000000000000000),
 ( 1.000000000000000000, 0.7866813202764355584, 1.000000000000000000),
 ( 1.000000000000000000, 0.7921509987295953792, 1.000000000000000000),
 ( 1.000000000000000000, 0.7948100380742536553, 1.000000000000000000),
 ( 1.000000000000000000, 0.8023666703953391544, 1.000000000000000000),
 ( 1.000000000000000000, 0.8068432255863590141, 1.000000000000000000),
 ( 1.000000000000000000, 0.8126963150101803590, 1.000000000000000000),
 ( 1.000000000000000000, 0.8145123882373950241, 1.000000000000000000),
 ( 1.000000000000000000, 0.8177588193891505153, 1.000000000000000000),
 ( 1.000000000000000000, 0.8191832667250861233, 1.000000000000000000),
 ( 1.000000000000000000, 0.8228396104941044786, 1.000000000000000000),
 ( 1.000000000000000000, 0.8244610879124180114, 1.000000000000000000),
 ( 1.000000000000000000, 0.8250833044923667758, 1.000000000000000000) ) ) 
 REPRESENTATION_ITEM ( '' )  SURFACE ( )  );
#12562=DIRECTION ( 'NONE',  ( 0.000000000000000000, 0.000000000000000000, 1.000000000000000000 ) ) ;
#12582=DIRECTION ( 'NONE',  ( 0.000000000000000000, 0.000000000000000000, 1.000000000000000000 ) ) ;
#12585=CARTESIAN_POINT ( 'NONE',  ( 13.78187932340991217, -67.90279320104012584, 3.641642753176146829 ) ) ;
#12587=CARTESIAN_POINT ( 'NONE',  ( 32.57431034208369880, -53.70580518431705741, -2.277903996697544731 ) ) ;
#12607=AXIS2_PLACEMENT_3D ( 'NONE', #7407, #9658, #259 ) ;
#12610=CARTESIAN_POINT ( 'NONE',  ( 9.430346510207451516, -54.59388862152623290, -3.160229925968730758 ) ) ;
#12614=CARTESIAN_POINT ( 'NONE',  ( 33.12442989620986822, -59.21224831720010684, 1.832439066040445708 ) ) ;
#12615=EDGE_LOOP ( 'NONE', ( #7291, #10872 ) ) ;
#12622=EDGE_CURVE ( 'NONE', #8156, #10038, #5962, .T. ) ;
#12628=DIRECTION ( 'NONE',  ( 0.000000000000000000, 1.000000000000000000, 0.000000000000000000 ) ) ;
#12637=CARTESIAN_POINT ( 'NONE',  ( 27.81410232013309525, -66.06148843087626688, -4.401172203687827356 ) ) ;
#12646=DIRECTION ( 'NONE',  ( 0.000000000000000000, 0.000000000000000000, 1.000000000000000000 ) ) ;
#12649=ORIENTED_EDGE ( 'NONE', *, *, #14162, .F. ) ;
#12651=VERTEX_POINT ( 'NONE', #7656 ) ;
#12652=CARTESIAN_POINT ( 'NONE',  ( 29.70251902843243741, -52.24929059928630437, -4.175384597093465544 ) ) ;
#12654=ORIENTED_EDGE ( 'NONE', *, *, #12622, .T. ) ;
#12657=B_SPLINE_CURVE_WITH_KNOTS ( 'NONE', 3,
 ( #6715, #783, #14793, #13793, #11399, #14869, #5566, #5645, #4561, #10337, #1015, #5735, #15032, #10261, #4484, #7798, #12491, #4247 ),
 .UNSPECIFIED., .F., .F.,
 ( 4, 2, 2, 2, 2, 2, 2, 2, 4 ),
 ( 0.000000000000000000, 0.0007591815323294819756, 0.001518363064658963951, 0.002277544596988445493, 0.003036726129317927902, 0.003795907661647409878, 0.004555089193976890986, 0.005314270726306382503, 0.006073452258635873152 ),
 .UNSPECIFIED. ) ;
#12663=CARTESIAN_POINT ( 'NONE',  ( 32.43636434651678258, -59.39117099671923228, 2.764779704643939073 ) ) ;
#12666=DIRECTION ( 'NONE',  ( -0.000000000000000000, 1.000000000000000000, -0.000000000000000000 ) ) ;
#12668=CARTESIAN_POINT ( 'NONE',  ( 6.635030218769952803, -47.02811197266219523, -2.732446379177816187 ) ) ;
#12679=ORIENTED_EDGE ( 'NONE', *, *, #881, .T. ) ;
#12683=CARTESIAN_POINT ( 'NONE',  ( 8.201103799357261082, -57.48563641131178770, -1.816685854991394455 ) ) ;
#12701=FACE_OUTER_BOUND ( 'NONE', #1410, .T. ) ;
#12704=AXIS2_PLACEMENT_3D ( 'NONE', #7517, #11268, #14520 ) ;
#12705=ADVANCED_FACE ( 'NONE', ( #14725 ), #4026, .T. ) ;
#12707=CARTESIAN_POINT ( 'NONE',  ( 29.14554934997181590, -50.05638191677163462, 4.212312498554270590 ) ) ;
#12716=DIRECTION ( 'NONE',  ( -0.000000000000000000, -0.000000000000000000, -1.000000000000000000 ) ) ;
#12728=CARTESIAN_POINT ( 'NONE',  ( 11.11753584644737280, -62.41236107492795782, 2.580051240451665784 ) ) ;
#12735=CARTESIAN_POINT ( 'NONE',  ( 27.84032651173070860, -68.65142943889377136, -4.053691724355999781 ) ) ;
#12737=ORIENTED_EDGE ( 'NONE', *, *, #10358, .F. ) ;
#12739=CARTESIAN_POINT ( 'NONE',  ( 11.81201825756313539, -52.27654955159783157, 3.048121150676241786 ) ) ;
#12745=CARTESIAN_POINT ( 'NONE',  ( 13.86157779355430186, -69.45278782524461292, 3.616934341765148719 ) ) ;
#12748=CARTESIAN_POINT ( 'NONE',  ( 31.99980918299992538, -53.15380395407657232, -2.455672049130702028 ) ) ;
#12750=EDGE_CURVE ( 'NONE', #4753, #15091, #7191, .T. ) ;
#12752=CARTESIAN_POINT ( 'NONE',  ( 9.236734562794072900, -59.22985212983980574, 2.757908476812879872 ) ) ;
#12755=B_SPLINE_CURVE_WITH_KNOTS ( 'NONE', 3,
 ( #5465, #10159, #6898, #15137, #12458, #6386, #13985, #1914 ),
 .UNSPECIFIED., .F., .F.,
 ( 4, 2, 2, 4 ),
 ( 0.000000000000000000, 0.0002685324218445792163, 0.0005370648436891596253, 0.001074129687378317299 ),
 .UNSPECIFIED. ) ;
#12764=CARTESIAN_POINT ( 'NONE',  ( 16.17808712815840266, -52.24929059925523234, -5.670202843295511386 ) ) ;
#12767=CARTESIAN_POINT ( 'NONE',  ( 10.00121363803638808, -52.94991738523399505, -2.538129127158726739 ) ) ;
#12768=DIRECTION ( 'NONE',  ( 0.000000000000000000, -0.000000000000000000, 1.000000000000000000 ) ) ;
#12771=VERTEX_POINT ( 'NONE', #6280 ) ;
#12773=EDGE_CURVE ( 'NONE', #7237, #8156, #14315, .T. ) ;
#12779=VERTEX_POINT ( 'NONE', #11486 ) ;
#12781=CARTESIAN_POINT ( 'NONE',  ( 23.10474973039555735, -53.24929059928630437, 5.564967562786288902 ) ) ;
#12785=CARTESIAN_POINT ( 'NONE',  ( 8.990236908599356980, -55.34783937825962141, -2.956317232382419835 ) ) ;
#12790=CARTESIAN_POINT ( 'NONE',  ( 25.54537353428280611, -52.24929059928630437, 5.670202843357490252 ) ) ;
#12791=CARTESIAN_POINT ( 'NONE',  ( 24.27245784421982222, -72.28366650276025496, 6.113054590620157214 ) ) ;
#12793=CARTESIAN_POINT ( 'NONE',  ( 20.86173033120691045, -53.24929059928630437, 6.000000000000000000 ) ) ;
#12816=CARTESIAN_POINT ( 'NONE',  ( 8.987770063152476396, -53.89143413596318055, 2.226202503535223531 ) ) ;
#12821=EDGE_CURVE ( 'NONE', #8129, #6079, #11789, .T. ) ;
#12834=ORIENTED_EDGE ( 'NONE', *, *, #5411, .T. ) ;
#12839=ORIENTED_EDGE ( 'NONE', *, *, #8938, .F. ) ;
#12847=ADVANCED_FACE ( 'NONE', ( #8957 ), #14801, .F. ) ;
#12850=CARTESIAN_POINT ( 'NONE',  ( 9.159236525127615991, -55.01088356445123395, -3.038469202939837466 ) ) ;
#12855=CARTESIAN_POINT ( 'NONE',  ( 33.12582565096496978, -59.20619211347772648, 2.502190571104487393 ) ) ;
#12856=VERTEX_POINT ( 'NONE', #13884 ) ;
#12857=CARTESIAN_POINT ( 'NONE',  ( 13.47393939923805561, -64.89111109908232322, 4.244693487287860556 ) ) ;
#12865=AXIS2_PLACEMENT_3D ( 'NONE', #3234, #11456, #7937 ) ;
#12873=CARTESIAN_POINT ( 'NONE',  ( 29.35555050496136076, -52.24929059928630437, 3.199931146564416462 ) ) ;
#12877=CARTESIAN_POINT ( 'NONE',  ( 18.61871093201826000, -52.24929059928630437, 5.564967562786272914 ) ) ;
#12885=CARTESIAN_POINT ( 'NONE',  ( 31.72322230991231962, -61.42570632716525125, 2.132522520905362651 ) ) ;
#12890=CARTESIAN_POINT ( 'NONE',  ( 32.36512860216036103, -60.82697974174514144, -1.965378744864697103 ) ) ;
#12891=CARTESIAN_POINT ( 'NONE',  ( 9.369695877296390307, -60.81027516727737492, 1.970305681586464130 ) ) ;
#12907=CARTESIAN_POINT ( 'NONE',  ( 13.86173033120690334, -69.39711819508848123, 3.801276035476828685 ) ) ;
#12908=CARTESIAN_POINT ( 'NONE',  ( 31.69392142191828299, -52.92218391219104490, 3.457912412235188082 ) ) ;
#12909=EDGE_CURVE ( 'NONE', #4896, #10195, #853, .T. ) ;
#12911=EDGE_CURVE ( 'NONE', #6655, #9231, #14810, .T. ) ;
#12912=EDGE_CURVE ( 'NONE', #8264, #5832, #9587, .T. ) ;
#12915=CARTESIAN_POINT ( 'NONE',  ( 20.86173033120691045, -57.24929059928630437, -3.000000000000000888 ) ) ;
#12919=DIRECTION ( 'NONE',  ( 0.000000000000000000, 0.000000000000000000, 1.000000000000000000 ) ) ;
#12921=CARTESIAN_POINT ( 'NONE',  ( 12.03298173962126860, -53.28399145779480506, -4.141535524925034295 ) ) ;
#12927=EDGE_LOOP ( 'NONE', ( #6739, #8513, #883, #2301, #3633, #5746, #14196, #11000, #811, #14759, #12654, #14329 ) ) ;
#12928=CARTESIAN_POINT ( 'NONE',  ( 20.86173033120691045, -52.24929059928630437, 0.000000000000000000 ) ) ;
#12929=ORIENTED_EDGE ( 'NONE', *, *, #622, .F. ) ;
#12953=CARTESIAN_POINT ( 'NONE',  ( 8.466388902489056179, -58.63671300496882566, 1.826958383912698158 ) ) ;
#12954=CARTESIAN_POINT ( 'NONE',  ( 29.69047892279255407, -53.28399145779480506, -4.141535524925019196 ) ) ;
#12956=CARTESIAN_POINT ( 'NONE',  ( 32.44735717182409473, -60.71989949371816664, -2.646748467233224211 ) ) ;
#12962=AXIS2_PLACEMENT_3D ( 'NONE', #3109, #7813, #12273 ) ;
#12969=DIRECTION ( 'NONE',  ( 0.7546336727145946943, 0.5961293309129324092, -0.2741493039031500656 ) ) ;
#12971=ORIENTED_EDGE ( 'NONE', *, *, #8668, .T. ) ;
#12981=CARTESIAN_POINT ( 'NONE',  ( 9.982851463787662638, -60.49988549795173043, 2.962481358178291391 ) ) ;
#12983=CARTESIAN_POINT ( 'NONE',  ( 29.67025276671635936, -52.24929059928631148, 3.114169983390998375 ) ) ;
#12989=ORIENTED_EDGE ( 'NONE', *, *, #11289, .F. ) ;
#12995=CARTESIAN_POINT ( 'NONE',  ( 10.58727470799617087, -61.88944072237683258, -2.366779157396529332 ) ) ;
#12996=EDGE_CURVE ( 'NONE', #3720, #10536, #4710, .T. ) ;
#12998=CARTESIAN_POINT ( 'NONE',  ( 9.586149153331275485, -54.40375996999062380, 3.226241354721975263 ) ) ;
#13000=CARTESIAN_POINT ( 'NONE',  ( 20.86173033120691045, -57.24929059928630437, 0.000000000000000000 ) ) ;
#13001=DIRECTION ( 'NONE',  ( 0.000000000000000000, -1.000000000000000000, 0.000000000000000000 ) ) ;
#13036=CARTESIAN_POINT ( 'NONE',  ( 33.59652235677629051, -57.16383106728765284, 1.814529264940141662 ) ) ;
#13038=CARTESIAN_POINT ( 'NONE',  ( 29.69047892279255052, -53.28399145779481216, -4.141535524925020084 ) ) ;
#13043=CARTESIAN_POINT ( 'NONE',  ( 31.95882812935311179, -60.25800154558402255, -2.890242835725726600 ) ) ;
#13053=CARTESIAN_POINT ( 'NONE',  ( 32.50130901777686177, -54.90141807276702934, 3.067753764789294291 ) ) ;
#13063=( BOUNDED_SURFACE ( )  B_SPLINE_SURFACE ( 3, 2, ( 
 ( #3596, #6988, #4678 ),
 ( #3880, #8230, #1647 ),
 ( #9821, #2807, #67 ),
 ( #14147, #12184, #5921 ) ),
 .UNSPECIFIED., .F., .F., .F. ) 
 B_SPLINE_SURFACE_WITH_KNOTS ( ( 4, 4 ),
 ( 3, 3 ),
 ( 0.000000000000000000, 0.001771943201165739230 ),
 ( 0.000000000000000000, 1.000000000000000000 ),
 .UNSPECIFIED. ) 
 GEOMETRIC_REPRESENTATION_ITEM ( )  RATIONAL_B_SPLINE_SURFACE ( (
 ( 1.000000000000000000, 0.8250833044923664428, 1.000000000000000000),
 ( 1.000000000000000000, 0.8269348987755780200, 1.000000000000000000),
 ( 1.000000000000000000, 0.8288551047899420654, 1.000000000000000000),
 ( 1.000000000000000000, 0.8308543624379425285, 1.000000000000000000) ) ) 
 REPRESENTATION_ITEM ( '' )  SURFACE ( )  );
#13065=CARTESIAN_POINT ( 'NONE',  ( 12.06345512429583877, -63.57773214734889677, -2.964070158660714327 ) ) ;
#13078=CARTESIAN_POINT ( 'NONE',  ( 29.30348265400095542, -64.16417350152460131, 3.791131921651011538 ) ) ;
#13085=EDGE_CURVE ( 'NONE', #11311, #13981, #3252, .T. ) ;
#13092=CARTESIAN_POINT ( 'NONE',  ( 20.86173033120691045, -82.24929059928629727, 0.000000000000000000 ) ) ;
#13093=ORIENTED_EDGE ( 'NONE', *, *, #112, .T. ) ;
#13096=AXIS2_PLACEMENT_3D ( 'NONE', #7296, #6008, #146 ) ;
#13102=DIRECTION ( 'NONE',  ( -0.000000000000000000, -0.000000000000000000, -1.000000000000000000 ) ) ;
#13109=CARTESIAN_POINT ( 'NONE',  ( 6.986309121235717789, -48.72433491191959831, 2.732636121739603130 ) ) ;
#13111=LINE ( 'NONE', #14261, #10273 ) ;
#13115=CARTESIAN_POINT ( 'NONE',  ( 29.92873905722243322, -53.28554919726588679, -4.056729053556589193 ) ) ;
#13117=EDGE_LOOP ( 'NONE', ( #13477, #2987, #4912, #1569, #7500 ) ) ;
#13120=AXIS2_PLACEMENT_3D ( 'NONE', #8966, #7589, #2043 ) ;
#13129=CARTESIAN_POINT ( 'NONE',  ( 32.55554926572738594, -53.68459816487440861, 2.283893849732154369 ) ) ;
#13130=ORIENTED_EDGE ( 'NONE', *, *, #14267, .T. ) ;
#13131=DIRECTION ( 'NONE',  ( -0.000000000000000000, -1.000000000000000000, -0.000000000000000000 ) ) ;
#13142=CARTESIAN_POINT ( 'NONE',  ( 8.093541475047761224, -56.17545244456535869, 1.862977194133688341 ) ) ;
#13150=( BOUNDED_SURFACE ( )  B_SPLINE_SURFACE ( 3, 2, ( 
 ( #14663, #13431, #2896 ),
 ( #12431, #7593, #4118 ),
 ( #8813, #12283, #1736 ),
 ( #13512, #6436, #1817 ),
 ( #13664, #10053, #10133 ),
 ( #3053, #4267, #6507 ) ),
 .UNSPECIFIED., .F., .F., .F. ) 
 B_SPLINE_SURFACE_WITH_KNOTS ( ( 4, 2, 4 ),
 ( 3, 3 ),
 ( -9.757819552369539906E-18, 0.001008510999900088731, 0.002017021999800187437 ),
 ( 0.000000000000000000, 1.000000000000000000 ),
 .UNSPECIFIED. ) 
 GEOMETRIC_REPRESENTATION_ITEM ( )  RATIONAL_B_SPLINE_SURFACE ( (
 ( 1.000000000000000000, 0.8053615646146047302, 1.000000000000000000),
 ( 1.000000000000000000, 0.8146689552415620206, 1.000000000000000000),
 ( 1.000000000000000000, 0.8215765256473256395, 1.000000000000000000),
 ( 1.000000000000000000, 0.8301698670440428307, 1.000000000000000000),
 ( 1.000000000000000000, 0.8316880482409466646, 1.000000000000000000),
 ( 1.000000000000000000, 0.8308543624379426396, 1.000000000000000000) ) ) 
 REPRESENTATION_ITEM ( '' )  SURFACE ( )  );
#13153=CARTESIAN_POINT ( 'NONE',  ( 31.72322230991231962, -61.42570632716525125, 2.132522520905375973 ) ) ;
#13160=DIRECTION ( 'NONE',  ( 0.000000000000000000, -1.000000000000000000, 0.000000000000000000 ) ) ;
#13164=CYLINDRICAL_SURFACE ( 'NONE', #5998, 2.000000000000000000 ) ;
#13166=DIRECTION ( 'NONE',  ( 0.000000000000000000, -1.000000000000000000, 0.000000000000000000 ) ) ;
#13174=CARTESIAN_POINT ( 'NONE',  ( 27.60448374887417344, -53.27035328036003392, -4.884026039770254179 ) ) ;
#13183=CARTESIAN_POINT ( 'NONE',  ( 30.88646442064404241, -52.52046121080019248, -2.777687341764009332 ) ) ;
#13190=ORIENTED_EDGE ( 'NONE', *, *, #7814, .F. ) ;
#13192=ORIENTED_EDGE ( 'NONE', *, *, #3576, .T. ) ;
#13203=CARTESIAN_POINT ( 'NONE',  ( 18.61871093201827065, -53.24929059928630437, -5.564967562786291566 ) ) ;
#13217=AXIS2_PLACEMENT_3D ( 'NONE', #13203, #9597, #8364 ) ;
#13219=CARTESIAN_POINT ( 'NONE',  ( 8.599038152243162259, -54.47420853489223447, 2.874994438546353503 ) ) ;
#13228=B_SPLINE_CURVE_WITH_KNOTS ( 'NONE', 3,
 ( #13475, #4229, #764, #1703 ),
 .UNSPECIFIED., .F., .F.,
 ( 4, 4 ),
 ( 0.000000000000000000, 0.003645914952990592789 ),
 .UNSPECIFIED. ) ;
#13234=CARTESIAN_POINT ( 'NONE',  ( 29.87892709566704497, -63.30956378473970148, 2.875213255997512540 ) ) ;
#13238=DIRECTION ( 'NONE',  ( -0.000000000000000000, 1.000000000000000000, -0.000000000000000000 ) ) ;
#13243=ORIENTED_EDGE ( 'NONE', *, *, #3896, .T. ) ;
#13244=EDGE_CURVE ( 'NONE', #9663, #8444, #7843, .T. ) ;
#13247=ADVANCED_FACE ( 'NONE', ( #3605 ), #226, .F. ) ;
#13257=CARTESIAN_POINT ( 'NONE',  ( 31.89675648641932071, -61.28862151863886965, 2.085432713781510738 ) ) ;
#13260=CARTESIAN_POINT ( 'NONE',  ( 31.18383636339185827, -53.65556550047445228, -3.599583915703545411 ) ) ;
#13268=CARTESIAN_POINT ( 'NONE',  ( 8.821484763567294607, -57.33450387999030795, -2.749014434309871469 ) ) ;
#13272=EDGE_CURVE ( 'NONE', #13625, #12856, #14287, .T. ) ;
#13279=CARTESIAN_POINT ( 'NONE',  ( 28.78915391981847804, -54.56989982938152650, -4.214561585076694428 ) ) ;
#13281=EDGE_CURVE ( 'NONE', #10908, #2336, #11135, .T. ) ;
#13287=DIRECTION ( 'NONE',  ( 0.9274945937977119303, -6.485030681406579288E-16, 0.3738365665314423159 ) ) ;
#13291=DIRECTION ( 'NONE',  ( -0.2245701561649801337, 0.9744137433416110161, 0.009279102705852840596 ) ) ;
#13298=CARTESIAN_POINT ( 'NONE',  ( 31.27094208184040625, -61.76394201827576325, 3.065891788227224080 ) ) ;
#13302=DIRECTION ( 'NONE',  ( -0.000000000000000000, 1.000000000000000000, -0.000000000000000000 ) ) ;
#13306=AXIS2_PLACEMENT_3D ( 'NONE', #4121, #6509, #8817 ) ;
#13314=EDGE_LOOP ( 'NONE', ( #12553, #14391, #14649, #3374, #1440, #11365, #3057, #2588, #12040 ) ) ;
#13324=ADVANCED_FACE ( 'NONE', ( #2825 ), #9982, .F. ) ;
#13331=CARTESIAN_POINT ( 'NONE',  ( 13.51972775594646770, -66.75404937493283342, -3.551013195542459311 ) ) ;
#13332=AXIS2_PLACEMENT_3D ( 'NONE', #11158, #14616, #2928 ) ;
#13333=AXIS2_PLACEMENT_3D ( 'NONE', #4691, #9393, #10617 ) ;
#13339=CARTESIAN_POINT ( 'NONE',  ( 8.948125790170781357, -57.91121052158847959, -2.751677492798585423 ) ) ;
#13340=CARTESIAN_POINT ( 'NONE',  ( 33.38971411695204949, -58.06117555224668081, -1.821720187976995975 ) ) ;
#13357=EDGE_CURVE ( 'NONE', #143, #2517, #15055, .T. ) ;
#13359=CARTESIAN_POINT ( 'NONE',  ( 10.83699624176960619, -52.52046121080027774, 2.777687341763831697 ) ) ;
#13365=DIRECTION ( 'NONE',  ( -0.000000000000000000, 1.000000000000000000, 0.000000000000000000 ) ) ;
#13372=ORIENTED_EDGE ( 'NONE', *, *, #2739, .T. ) ;
#13376=CARTESIAN_POINT ( 'NONE',  ( 31.88156390563088749, -61.30062302791112927, -2.840369378987770421 ) ) ;
#13384=ORIENTED_EDGE ( 'NONE', *, *, #6088, .F. ) ;
#13385=CARTESIAN_POINT ( 'NONE',  ( 31.89712467290438269, -61.28833066657261952, -2.085332803602909291 ) ) ;
#13388=DIRECTION ( 'NONE',  ( -0.000000000000000000, -0.000000000000000000, -1.000000000000000000 ) ) ;
#13390=CARTESIAN_POINT ( 'NONE',  ( 18.24879706501207721, -53.10810670090265262, 6.494041865157049287 ) ) ;
#13404=CARTESIAN_POINT ( 'NONE',  ( 9.834282440617473142, -54.14192065903538520, 3.328125142887254029 ) ) ;
#13408=EDGE_CURVE ( 'NONE', #3440, #14689, #2339, .T. ) ;
#13412=CARTESIAN_POINT ( 'NONE',  ( 17.09549820959326638, -85.24929059928631148, -1.347403282660980528 ) ) ;
#13418=CARTESIAN_POINT ( 'NONE',  ( 13.92166289842272597, -69.39711819508849544, -3.972674503026252246 ) ) ;
#13423=CARTESIAN_POINT ( 'NONE',  ( 10.12753145436369451, -53.91129217357575953, 3.442845340291940559 ) ) ;
#13425=CARTESIAN_POINT ( 'NONE',  ( 14.38963276113423895, -69.39711819508849544, 4.502057496415707405 ) ) ;
#13431=CARTESIAN_POINT ( 'NONE',  ( 9.841896756782944067, -61.30062302791112927, 2.840369378987773530 ) ) ;
#13436=CARTESIAN_POINT ( 'NONE',  ( 27.67989258697498300, -66.53205946168893092, 4.446982897616673647 ) ) ;
#13441=CARTESIAN_POINT ( 'NONE',  ( 33.25875691633515174, -58.62940108252875149, 2.501915095544871459 ) ) ;
#13446=CARTESIAN_POINT ( 'NONE',  ( 29.73572575534737794, -63.50313342086874968, -3.632148419035127418 ) ) ;
#13448=ORIENTED_EDGE ( 'NONE', *, *, #13590, .F. ) ;
#13450=CARTESIAN_POINT ( 'NONE',  ( 29.35555050496136431, -52.24929059928631148, 3.199931146564417350 ) ) ;
#13469=CARTESIAN_POINT ( 'NONE',  ( 8.766382814749736241, -57.08357682498793650, -2.747855728347990745 ) ) ;
#13475=CARTESIAN_POINT ( 'NONE',  ( 17.61519226005271577, -69.39711819508849544, 6.201611931792121446 ) ) ;
#13476=CARTESIAN_POINT ( 'NONE',  ( 13.78187932340991040, -67.90279320104012584, -3.641642753162454671 ) ) ;
#13477=ORIENTED_EDGE ( 'NONE', *, *, #1694, .T. ) ;
#13479=CARTESIAN_POINT ( 'NONE',  ( 20.86173033120691045, -69.39711819508849544, 0.000000000000000000 ) ) ;
#13481=DIRECTION ( 'NONE',  ( 0.000000000000000000, 0.000000000000000000, 1.000000000000000000 ) ) ;
#13483=ORIENTED_EDGE ( 'NONE', *, *, #4166, .T. ) ;
#13488=DIRECTION ( 'NONE',  ( 0.000000000000000000, -1.000000000000000000, 0.000000000000000000 ) ) ;
#13492=ORIENTED_EDGE ( 'NONE', *, *, #12153, .T. ) ;
#13503=VECTOR ( 'NONE', #13698, 1000.000000000000000 ) ;
#13504=EDGE_CURVE ( 'NONE', #14689, #6655, #658, .T. ) ;
#13507=CARTESIAN_POINT ( 'NONE',  ( 9.505449653674235222, -53.34475964609201526, 2.389227176380498641 ) ) ;
#13510=AXIS2_PLACEMENT_3D ( 'NONE', #9736, #3864, #7413 ) ;
#13512=CARTESIAN_POINT ( 'NONE',  ( 9.399792925529615317, -59.70501925844563118, 2.784164790581823645 ) ) ;
#13522=DIRECTION ( 'NONE',  ( 0.000000000000000000, 1.000000000000000000, 0.000000000000000000 ) ) ;
#13523=ORIENTED_EDGE ( 'NONE', *, *, #13408, .F. ) ;
#13536=EDGE_CURVE ( 'NONE', #9144, #8129, #5837, .T. ) ;
#13545=EDGE_CURVE ( 'NONE', #3720, #1828, #9689, .T. ) ;
#13549=ORIENTED_EDGE ( 'NONE', *, *, #6325, .T. ) ;
#13551=CARTESIAN_POINT ( 'NONE',  ( 33.59512494182110487, -55.93948076112101120, 2.601440957439760115 ) ) ;
#13571=ORIENTED_EDGE ( 'NONE', *, *, #13638, .T. ) ;
#13572=CARTESIAN_POINT ( 'NONE',  ( 23.47858629692700561, -53.24929059928630437, -6.492462156583982846 ) ) ;
#13577=VERTEX_POINT ( 'NONE', #12915 ) ;
#13580=CARTESIAN_POINT ( 'NONE',  ( 12.41997800841365773, -64.16417350152165966, 3.791131921655388037 ) ) ;
#13582=CARTESIAN_POINT ( 'NONE',  ( 33.48164203564194707, -55.39134602458726420, -1.947764125980440797 ) ) ;
#13590=EDGE_CURVE ( 'NONE', #12406, #10773, #10852, .T. ) ;
#13592=CARTESIAN_POINT ( 'NONE',  ( 8.091875466796993877, -56.84741961274605160, 1.823451407584537609 ) ) ;
#13596=B_SPLINE_CURVE_WITH_KNOTS ( 'NONE', 3,
 ( #7137, #8139, #6986, #9452, #8062, #3363 ),
 .UNSPECIFIED., .F., .F.,
 ( 4, 2, 4 ),
 ( 0.001000432843099107122, 0.009082381923694659437, 0.01716433100429023278 ),
 .UNSPECIFIED. ) ;
#13597=B_SPLINE_CURVE_WITH_KNOTS ( 'NONE', 3,
 ( #13425, #13896, #7126, #2431, #8213, #9441, #12907, #1200 ),
 .UNSPECIFIED., .F., .F.,
 ( 4, 2, 2, 4 ),
 ( 0.000000000000000000, 0.0002685268308981082351, 0.0005370536617962164702, 0.001074107323592430338 ),
 .UNSPECIFIED. ) ;
#13600=DIRECTION ( 'NONE',  ( -0.000000000000000000, 1.000000000000000000, -0.000000000000000000 ) ) ;
#13617=CARTESIAN_POINT ( 'NONE',  ( 8.700745695602643437, -59.65359113318982054, -1.835578343538661672 ) ) ;
#13622=CARTESIAN_POINT ( 'NONE',  ( 32.98169228882561299, -56.83327624868833539, -2.758240060640952951 ) ) ;
#13624=CARTESIAN_POINT ( 'NONE',  ( 12.66974950169169567, -64.60713873539394569, -3.212402267258147592 ) ) ;
#13625=VERTEX_POINT ( 'NONE', #7049 ) ;
#13631=( BOUNDED_SURFACE ( )  B_SPLINE_SURFACE ( 3, 2, ( 
 ( #11404, #4408, #2183 ),
 ( #7962, #6794, #9112 ),
 ( #9031, #11482, #8113 ),
 ( #15038, #12495, #4490 ),
 ( #1942, #6875, #13726 ),
 ( #11560, #4252, #6958 ) ),
 .UNSPECIFIED., .F., .F., .F. ) 
 B_SPLINE_SURFACE_WITH_KNOTS ( ( 4, 2, 4 ),
 ( 3, 3 ),
 ( 1.084202172485504434E-19, 0.001005789800061012871, 0.002011579600122025743 ),
 ( 0.000000000000000000, 1.000000000000000000 ),
 .UNSPECIFIED. ) 
 GEOMETRIC_REPRESENTATION_ITEM ( )  RATIONAL_B_SPLINE_SURFACE ( (
 ( 1.000000000000000000, 0.8308543624379417514, 1.000000000000000000),
 ( 1.000000000000000000, 0.8317114229144060289, 1.000000000000000000),
 ( 1.000000000000000000, 0.8301458553065871326, 1.000000000000000000),
 ( 1.000000000000000000, 0.8215594255318671157, 1.000000000000000000),
 ( 1.000000000000000000, 0.8147253674582816130, 1.000000000000000000),
 ( 1.000000000000000000, 0.8053615646146046192, 1.000000000000000000) ) ) 
 REPRESENTATION_ITEM ( '' )  SURFACE ( )  );
#13638=EDGE_CURVE ( 'NONE', #9843, #9144, #8726, .T. ) ;
#13639=FACE_OUTER_BOUND ( 'NONE', #6242, .T. ) ;
#13642=CYLINDRICAL_SURFACE ( 'NONE', #1513, 3.000000000000000888 ) ;
#13648=CARTESIAN_POINT ( 'NONE',  ( 8.538156564172162177, -54.60220113588928115, 2.070297547960220808 ) ) ;
#13656=CARTESIAN_POINT ( 'NONE',  ( 8.890669559332980754, -60.05631636466448953, -1.868376189747823046 ) ) ;
#13658=CARTESIAN_POINT ( 'NONE',  ( 11.13121913594275370, -52.42016302384273985, 2.859972208322074660 ) ) ;
#13659=CARTESIAN_POINT ( 'NONE',  ( 33.26342499051592938, -54.78204083127141644, -2.039726671434834770 ) ) ;
#13661=CARTESIAN_POINT ( 'NONE',  ( 25.18496984658901638, -69.39711819508849544, 5.637959728397568426 ) ) ;
#13664=CARTESIAN_POINT ( 'NONE',  ( 9.273438744392825228, -59.39772283578258794, 2.758706911751842128 ) ) ;
#13667=ORIENTED_EDGE ( 'NONE', *, *, #14162, .T. ) ;
#13680=CARTESIAN_POINT ( 'NONE',  ( 8.090375438032983979, -56.83262086368637256, -1.823905708655537028 ) ) ;
#13695=CARTESIAN_POINT ( 'NONE',  ( 9.272883950264748876, -59.39518542680082192, -2.758694842813115056 ) ) ;
#13698=DIRECTION ( 'NONE',  ( -0.000000000000000000, -0.000000000000000000, -1.000000000000000000 ) ) ;
#13709=CARTESIAN_POINT ( 'NONE',  ( 24.18480965113672099, -70.79589105105083036, 6.161139702147667485 ) ) ;
#13721=DIRECTION ( 'NONE',  ( -0.000000000000000000, -1.000000000000000000, -0.000000000000000000 ) ) ;
#13726=CARTESIAN_POINT ( 'NONE',  ( 32.06857839880813543, -61.15288932781299991, 2.038807541295255543 ) ) ;
#13728=CARTESIAN_POINT ( 'NONE',  ( 25.54537353427514645, -52.24929059928631148, -5.670202843350166333 ) ) ;
#13731=ORIENTED_EDGE ( 'NONE', *, *, #9727, .F. ) ;
#13735=CARTESIAN_POINT ( 'NONE',  ( 13.12221348233057050, -65.57050171853551035, 4.044987206838578153 ) ) ;
#13744=CARTESIAN_POINT ( 'NONE',  ( 18.22133905414316501, -54.09900330348973085, -6.482993899727721221 ) ) ;
#13747=CARTESIAN_POINT ( 'NONE',  ( 32.64893527110322680, -58.48797006926987052, -2.754379914540423968 ) ) ;
#13749=VERTEX_POINT ( 'NONE', #3886 ) ;
#13758=CARTESIAN_POINT ( 'NONE',  ( 9.782925212513372770, -53.09518070810211299, -3.364836540200758286 ) ) ;
#13766=VERTEX_POINT ( 'NONE', #14579 ) ;
#13767=EDGE_CURVE ( 'NONE', #7109, #12771, #14295, .T. ) ;
#13774=PLANE ( 'NONE',  #14673 ) ;
#13776=CARTESIAN_POINT ( 'NONE',  ( 29.69047892279255407, -53.28399145779480506, -4.141535524925019196 ) ) ;
#13778=CARTESIAN_POINT ( 'NONE',  ( 27.83979445996965296, -68.65220048136343678, 4.053998922580534625 ) ) ;
#13785=DIRECTION ( 'NONE',  ( -0.000000000000000000, 1.000000000000000000, -0.000000000000000000 ) ) ;
#13786=CARTESIAN_POINT ( 'NONE',  ( 33.52235686305655804, -57.48563641131178770, 2.500000000000000000 ) ) ;
#13793=CARTESIAN_POINT ( 'NONE',  ( 32.97418302199919538, -56.32592369292858336, 2.799485268159561890 ) ) ;
#13811=CARTESIAN_POINT ( 'NONE',  ( 32.87706978204689534, -54.07871170900528313, -2.179395260058141215 ) ) ;
#13815=AXIS2_PLACEMENT_3D ( 'NONE', #10115, #4256, #4494 ) ;
#13819=CARTESIAN_POINT ( 'NONE',  ( 12.57791131244190197, -50.05638191677160620, -4.212312498554237727 ) ) ;
#13833=EDGE_CURVE ( 'NONE', #7182, #7033, #4514, .T. ) ;
#13835=VERTEX_POINT ( 'NONE', #8514 ) ;
#13838=CARTESIAN_POINT ( 'NONE',  ( 9.122196393684426141, -53.72848551507318859, -3.102677277819655632 ) ) ;
#13840=DIRECTION ( 'NONE',  ( 0.000000000000000000, -1.000000000000000000, 0.000000000000000000 ) ) ;
#13843=CARTESIAN_POINT ( 'NONE',  ( 32.52281604437752804, -59.06479067038042530, 2.757123406423269696 ) ) ;
#13845=CARTESIAN_POINT ( 'NONE',  ( 9.175559494770812563, -57.26105658658105568, -1.816685854991390014 ) ) ;
#13852=CARTESIAN_POINT ( 'NONE',  ( 11.79136029199137958, -53.28557117198400306, -4.055532625545659187 ) ) ;
#13863=VERTEX_POINT ( 'NONE', #2811 ) ;
#13881=CARTESIAN_POINT ( 'NONE',  ( 27.87319062054570296, -68.05254135531041015, -4.069129117103200244 ) ) ;
#13882=ORIENTED_EDGE ( 'NONE', *, *, #12911, .F. ) ;
#13884=CARTESIAN_POINT ( 'NONE',  ( 33.12442989620986822, -59.21224831720011395, 1.832439066039631914 ) ) ;
#13890=B_SPLINE_CURVE_WITH_KNOTS ( 'NONE', 3,
 ( #6483, #12331, #11172, #2859 ),
 .UNSPECIFIED., .F., .F.,
 ( 4, 4 ),
 ( 0.006832557018188310620, 0.007799362039380771001 ),
 .UNSPECIFIED. ) ;
#13896=CARTESIAN_POINT ( 'NONE',  ( 14.30960301864961615, -69.39711819508850965, 4.459166325353795202 ) ) ;
#13899=CARTESIAN_POINT ( 'NONE',  ( 18.10076659936878585, -57.98711502975817211, -6.432599168430029657 ) ) ;
#13900=VERTEX_POINT ( 'NONE', #792 ) ;
#13906=CARTESIAN_POINT ( 'NONE',  ( 12.48148056143272377, -64.22824823034756037, -3.135769320951040218 ) ) ;
#13909=CARTESIAN_POINT ( 'NONE',  ( 9.025447862944712796, -53.84541978742826274, -3.062363702219679684 ) ) ;
#13913=ORIENTED_EDGE ( 'NONE', *, *, #6926, .F. ) ;
#13933=CARTESIAN_POINT ( 'NONE',  ( 33.50710080144106229, -55.48278564389710965, -2.668166895089373991 ) ) ;
#13936=CARTESIAN_POINT ( 'NONE',  ( 33.43530366116245744, -55.00412896308922939, 2.731447707963691851 ) ) ;
#13940=ADVANCED_FACE ( 'NONE', ( #8876 ), #4696, .T. ) ;
#13952=CARTESIAN_POINT ( 'NONE',  ( 33.12442989620986822, -59.21224831720009263, -1.832439066040486120 ) ) ;
#13955=CARTESIAN_POINT ( 'NONE',  ( 10.00023835250150483, -61.42570632716525125, 2.132522520905371977 ) ) ;
#13956=DIRECTION ( 'NONE',  ( 1.000000000000000000, 0.000000000000000000, -0.000000000000000000 ) ) ;
#13964=CARTESIAN_POINT ( 'NONE',  ( 20.86173033120691045, -82.24929059928629727, -3.999999999999999112 ) ) ;
#13965=CARTESIAN_POINT ( 'NONE',  ( 9.567742742854477456, -53.28162808095388669, 2.408690284354809030 ) ) ;
#13970=EDGE_CURVE ( 'NONE', #13900, #13577, #14532, .T. ) ;
#13973=LINE ( 'NONE', #7124, #4883 ) ;
#13979=CARTESIAN_POINT ( 'NONE',  ( 9.615492529877293748, -61.48517313030954057, -2.719255632331072370 ) ) ;
#13981=VERTEX_POINT ( 'NONE', #2101 ) ;
#13985=CARTESIAN_POINT ( 'NONE',  ( 27.49389128939799676, -69.39711819508849544, 4.416273062436605557 ) ) ;
#13987=EDGE_CURVE ( 'NONE', #12651, #5130, #3957, .T. ) ;
#13988=CARTESIAN_POINT ( 'NONE',  ( 16.19211320117534214, -53.25924031079298260, -5.665074923594194622 ) ) ;
#13991=CARTESIAN_POINT ( 'NONE',  ( 11.09435930935936554, -53.42013688713559816, -3.804487959019770216 ) ) ;
#14005=DIRECTION ( 'NONE',  ( 0.3738365665314423159, 0.000000000000000000, 0.9274945937977119303 ) ) ;
#14011=VERTEX_POINT ( 'NONE', #13964 ) ;
#14026=CARTESIAN_POINT ( 'NONE',  ( 31.88156390563087683, -61.30062302791112927, -2.840369378987771753 ) ) ;
#14028=CIRCLE ( 'NONE', #10803, 3.999999999999999112 ) ;
#14037=VECTOR ( 'NONE', #10355, 1000.000000000000000 ) ;
#14040=CARTESIAN_POINT ( 'NONE',  ( 11.27557984327373575, -52.38203995748321518, -2.900057921394206151 ) ) ;
#14047=DIRECTION ( 'NONE',  ( 0.000000000000000000, 1.000000000000000000, 0.000000000000000000 ) ) ;
#14051=CARTESIAN_POINT ( 'NONE',  ( 23.36173033120691400, -82.24929059928629727, 6.000000000000001776 ) ) ;
#14053=CARTESIAN_POINT ( 'NONE',  ( 32.05473995880635840, -54.31361072226614084, 3.260388240305548191 ) ) ;
#14055=CARTESIAN_POINT ( 'NONE',  ( 9.496763888311855695, -60.90158242453190951, -2.720958400102891250 ) ) ;
#14062=B_SPLINE_CURVE_WITH_KNOTS ( 'NONE', 3,
 ( #1929, #1852, #1785, #773, #7637, #14709, #14859, #11243, #4238, #12637, #849, #4162, #5488, #3244 ),
 .UNSPECIFIED., .F., .F.,
 ( 4, 2, 2, 2, 2, 2, 4 ),
 ( 8.673617379884035472E-19, 0.002516897397286764395, 0.003775346095930138136, 0.005033794794573512310, 0.006292243493216886051, 0.007550692191860259792, 0.01006758958914700727 ),
 .UNSPECIFIED. ) ;
#14066=CARTESIAN_POINT ( 'NONE',  ( 12.02094163398139770, -52.24929059928630437, -4.175384597093463768 ) ) ;
#14074=EDGE_CURVE ( 'NONE', #3807, #14139, #6004, .T. ) ;
#14087=AXIS2_PLACEMENT_3D ( 'NONE', #9832, #8727, #14512 ) ;
#14094=EDGE_CURVE ( 'NONE', #9073, #3836, #14119, .T. ) ;
#14119=LINE ( 'NONE', #8275, #9391 ) ;
#14133=CARTESIAN_POINT ( 'NONE',  ( 32.21946295013410122, -53.34604504765228938, 2.388784160329073814 ) ) ;
#14139=VERTEX_POINT ( 'NONE', #2717 ) ;
#14141=ORIENTED_EDGE ( 'NONE', *, *, #9176, .T. ) ;
#14144=( BOUNDED_SURFACE ( )  B_SPLINE_SURFACE ( 3, 2, ( 
 ( #5416, #12187, #4023 ),
 ( #567, #10968, #2728 ),
 ( #8797, #4098, #1720 ),
 ( #11181, #8718, #2959 ),
 ( #7652, #13279, #5119 ),
 ( #6277, #1864, #12122 ),
 ( #1801, #420, #7573 ),
 ( #6492, #5269, #9823 ),
 ( #12266, #632, #5340 ),
 ( #9964, #3950, #8649 ),
 ( #10190, #10342, #4568 ),
 ( #8954, #867, #3335 ),
 ( #7881, #13881, #10426 ),
 ( #15117, #12735, #9197 ) ),
 .UNSPECIFIED., .F., .F., .F. ) 
 B_SPLINE_SURFACE_WITH_KNOTS ( ( 4, 2, 2, 2, 2, 2, 4 ),
 ( 3, 3 ),
 ( 0.2948322565876199119, 0.2981287057529276030, 0.3014251549182353496, 0.3080180532488507872, 0.3146109515794662803, 0.3179074007447739714, 0.3212038499100817179 ),
 ( 0.000000000000000000, 0.9256633218932677210 ),
 .UNSPECIFIED. ) 
 GEOMETRIC_REPRESENTATION_ITEM ( )  RATIONAL_B_SPLINE_SURFACE ( (
 ( 1.000000000000000000, 0.9979219307738474987, 0.9996910464737041035),
 ( 1.000000000000000000, 0.9979571442240253720, 0.9996962817755257191),
 ( 1.000000000000000000, 0.9979896195972790540, 0.9997011099982617832),
 ( 1.000000000000000000, 0.9980478678146850191, 0.9997097699562369488),
 ( 1.000000000000000000, 0.9980736641738252590, 0.9997136051875283869),
 ( 1.000000000000000000, 0.9981411222207057232, 0.9997236344017617071),
 ( 1.000000000000000000, 0.9981728461537401342, 0.9997283509053582762),
 ( 1.000000000000000000, 0.9982102196780588965, 0.9997339073526521069),
 ( 1.000000000000000000, 0.9982158677593770957, 0.9997347470718578322),
 ( 1.000000000000000000, 0.9982052731646248178, 0.9997331719378983461),
 ( 1.000000000000000000, 0.9981985596398339489, 0.9997321738156357274),
 ( 1.000000000000000000, 0.9981789131846819929, 0.9997292529112105086),
 ( 1.000000000000000000, 0.9981660722458856050, 0.9997273438057427963),
 ( 1.000000000000000000, 0.9981504490785558792, 0.9997250210570212126) ) ) 
 REPRESENTATION_ITEM ( '' )  SURFACE ( )  );
#14146=CARTESIAN_POINT ( 'NONE',  ( 8.996939472011559857, -55.34955111272346784, 2.958349455637744541 ) ) ;
#14147=CARTESIAN_POINT ( 'NONE',  ( 9.200644618036294631, -59.06479067038042530, -2.757123406423244383 ) ) ;
#14156=CARTESIAN_POINT ( 'NONE',  ( 16.17808712816582783, -52.24929059928630437, 5.670202843280253369 ) ) ;
#14162=EDGE_CURVE ( 'NONE', #14011, #10151, #5448, .T. ) ;
#14169=DIRECTION ( 'NONE',  ( 0.000000000000000000, -1.000000000000000000, 0.000000000000000000 ) ) ;
#14182=FACE_OUTER_BOUND ( 'NONE', #12927, .T. ) ;
#14189=CARTESIAN_POINT ( 'NONE',  ( 33.44446161014174379, -55.23290567775144666, 1.966731800905200833 ) ) ;
#14191=CARTESIAN_POINT ( 'NONE',  ( 33.31720230358228463, -54.90785108970916184, -2.018552575027052765 ) ) ;
#14192=CIRCLE ( 'NONE', #5582, 3.999999999999999112 ) ;
#14196=ORIENTED_EDGE ( 'NONE', *, *, #2754, .T. ) ;
#14197=CARTESIAN_POINT ( 'NONE',  ( 8.091875466796944139, -56.52532528994184702, -1.842181053809134994 ) ) ;
#14199=CIRCLE ( 'NONE', #704, 0.9999999999999991118 ) ;
#14210=CARTESIAN_POINT ( 'NONE',  ( 32.56422413728613918, -55.01088356445131211, 3.038469202939856562 ) ) ;
#14211=EDGE_LOOP ( 'NONE', ( #2560, #6481, #15058, #11980 ) ) ;
#14214=ORIENTED_EDGE ( 'NONE', *, *, #6815, .F. ) ;
#14222=CARTESIAN_POINT ( 'NONE',  ( 9.277478075084694353, -53.56578013995677168, 2.318572182806073023 ) ) ;
#14223=EDGE_CURVE ( 'NONE', #9231, #4765, #14062, .T. ) ;
#14238=EDGE_LOOP ( 'NONE', ( #427, #14833, #2010, #12839 ) ) ;
#14239=CARTESIAN_POINT ( 'NONE',  ( 27.25620696618383221, -52.24929059928630437, -3.946667064627065180 ) ) ;
#14249=EDGE_CURVE ( 'NONE', #1508, #1111, #8890, .T. ) ;
#14261=CARTESIAN_POINT ( 'NONE',  ( 20.86173033120691045, -96.56299909827106376, -3.999999999999999112 ) ) ;
#14262=CARTESIAN_POINT ( 'NONE',  ( 27.80982499094064408, -66.07496666188232837, 4.402666029760359478 ) ) ;
#14265=CARTESIAN_POINT ( 'NONE',  ( 32.13731150908262180, -54.40375996999018327, -3.226241354721974819 ) ) ;
#14267=EDGE_CURVE ( 'NONE', #7109, #9216, #11465, .T. ) ;
#14268=CARTESIAN_POINT ( 'NONE',  ( 9.200644618036296407, -59.06479067038043240, -2.757123406423053424 ) ) ;
#14269=ORIENTED_EDGE ( 'NONE', *, *, #753, .T. ) ;
#14281=CARTESIAN_POINT ( 'NONE',  ( 29.97935572506992230, -52.28363178956111312, 3.029531835800513218 ) ) ;
#14287=CIRCLE ( 'NONE', #13096, 1.000000000000001110 ) ;
#14293=CARTESIAN_POINT ( 'NONE',  ( 8.872946762439195112, -55.70527662866908969, 2.889323894642001012 ) ) ;
#14295=CIRCLE ( 'NONE', #9133, 31.00000000000000000 ) ;
#14298=EDGE_LOOP ( 'NONE', ( #9285, #10845, #12246, #7304, #11501, #4529, #13667 ) ) ;
#14300=ORIENTED_EDGE ( 'NONE', *, *, #3154, .T. ) ;
#14306=CARTESIAN_POINT ( 'NONE',  ( 31.88156390563088038, -61.30062302791114348, 2.840369378987781968 ) ) ;
#14315=CIRCLE ( 'NONE', #10631, 3.999999999999999112 ) ;
#14321=DIRECTION ( 'NONE',  ( -0.000000000000000000, 1.000000000000000000, -0.000000000000000000 ) ) ;
#14329=ORIENTED_EDGE ( 'NONE', *, *, #9037, .T. ) ;
#14337=DIRECTION ( 'NONE',  ( 0.000000000000000000, 0.000000000000000000, -1.000000000000000000 ) ) ;
#14347=CARTESIAN_POINT ( 'NONE',  ( 33.33600117268625951, -54.92996021470965928, 2.012507329417090318 ) ) ;
#14350=ORIENTED_EDGE ( 'NONE', *, *, #1738, .F. ) ;
#14364=CARTESIAN_POINT ( 'NONE',  ( 29.93026052250974445, -53.28555914634976176, 4.056187502120626398 ) ) ;
#14377=CARTESIAN_POINT ( 'NONE',  ( 8.199792978590135561, -57.47994873761391688, 2.501453769636591495 ) ) ;
#14386=CARTESIAN_POINT ( 'NONE',  ( 30.71459926079626612, -62.29356353673582447, 3.270869388460270866 ) ) ;
#14391=ORIENTED_EDGE ( 'NONE', *, *, #15200, .T. ) ;
#14392=CARTESIAN_POINT ( 'NONE',  ( 29.10765984106734550, -64.50532980541194661, -3.862852061920468039 ) ) ;
#14394=EDGE_LOOP ( 'NONE', ( #8785, #6375, #946, #11833, #710, #14818, #1221, #12272, #1959 ) ) ;
#14402=ORIENTED_EDGE ( 'NONE', *, *, #12291, .T. ) ;
#14403=CARTESIAN_POINT ( 'NONE',  ( 12.36791015745245836, -56.52532528994181860, 2.500000000000000000 ) ) ;
#14417=CARTESIAN_POINT ( 'NONE',  ( 32.59950272815257222, -53.72645478541647890, -3.103403305059523554 ) ) ;
#14423=CARTESIAN_POINT ( 'NONE',  ( 33.25875691633304143, -58.62940108252828963, -2.501915095519685384 ) ) ;
#14446=PRODUCT_DEFINITION_FORMATION_WITH_SPECIFIED_SOURCE ( 'ANY', '', #7821, .NOT_KNOWN. ) ;
#14448=CARTESIAN_POINT ( 'NONE',  ( 8.256272429926839962, -55.33425260370182031, 2.693485533444373026 ) ) ;
#14452=LINE ( 'NONE', #8811, #12227 ) ;
#14456=ADVANCED_FACE ( 'NONE', ( #1392 ), #8407, .T. ) ;
#14461=CARTESIAN_POINT ( 'NONE',  ( 29.24098086411990849, -64.27177309650618042, 3.135762038895159698 ) ) ;
#14464=LINE ( 'NONE', #8471, #10493 ) ;
#14468=ORIENTED_EDGE ( 'NONE', *, *, #9886, .F. ) ;
#14483=EDGE_CURVE ( 'NONE', #10222, #8652, #12388, .T. ) ;
#14484=CARTESIAN_POINT ( 'NONE',  ( 12.65170711616557142, -50.97709764761836482, 4.214141842892688672 ) ) ;
#14487=CARTESIAN_POINT ( 'NONE',  ( 32.96955190781037004, -54.21180406361326476, -2.945963350965641769 ) ) ;
#14491=VERTEX_POINT ( 'NONE', #12239 ) ;
#14493=CARTESIAN_POINT ( 'NONE',  ( -12.09280073291247426, 0.000000000000000000, -11.78977872328358067 ) ) ;
#14501=CARTESIAN_POINT ( 'NONE',  ( 27.67348840388350339, -69.39711819508848123, -4.211076768700163342 ) ) ;
#14507=DIRECTION ( 'NONE',  ( 0.000000000000000000, 0.000000000000000000, -1.000000000000000000 ) ) ;
#14512=DIRECTION ( 'NONE',  ( 0.6198786537240922323, -0.7846976836063727090, 0.000000000000000000 ) ) ;
#14514=CARTESIAN_POINT ( 'NONE',  ( 53.81626139532630759, -82.24929059928629727, 11.78977872328355048 ) ) ;
#14516=DIRECTION ( 'NONE',  ( -1.000000000000000000, -0.000000000000000000, -0.000000000000000000 ) ) ;
#14520=DIRECTION ( 'NONE',  ( 0.000000000000000000, -0.000000000000000000, 1.000000000000000000 ) ) ;
#14525=CARTESIAN_POINT ( 'NONE',  ( 28.59185145675465733, -64.18054652438925700, 4.118450070758925996 ) ) ;
#14528=CARTESIAN_POINT ( 'NONE',  ( 8.821484763567294607, -57.33450387999030795, -2.749014434309871469 ) ) ;
#14532=CIRCLE ( 'NONE', #9876, 3.000000000000000888 ) ;
#14540=MANIFOLD_SOLID_BREP ( 'Fillet5', #11932 ) ;
#14544=EDGE_LOOP ( 'NONE', ( #5287, #672, #2457, #3990 ) ) ;
#14554=CARTESIAN_POINT ( 'NONE',  ( 9.841858720825518603, -62.60511169126380082, 2.715102820267620398 ) ) ;
#14564=CARTESIAN_POINT ( 'NONE',  ( 32.90197589884652274, -57.33450387999030085, -2.749014434309875909 ) ) ;
#14567=CARTESIAN_POINT ( 'NONE',  ( 33.52235686305655804, -57.48563641131178770, -1.816685854991392457 ) ) ;
#14569=CARTESIAN_POINT ( 'NONE',  ( 21.74884261173415467, -85.24929059928631148, -6.000000000000000888 ) ) ;
#14573=CARTESIAN_POINT ( 'NONE',  ( 28.56964104117922076, -65.59433601606471598, -3.409308316089457502 ) ) ;
#14579=CARTESIAN_POINT ( 'NONE',  ( 20.86173033120691045, -52.24929059928630437, 6.000000000000000000 ) ) ;
#14585=CARTESIAN_POINT ( 'NONE',  ( 11.55440981570039938, -53.31390540393576316, 3.970772651015708199 ) ) ;
#14594=CARTESIAN_POINT ( 'NONE',  ( 30.17008156804327612, -53.31401535610196163, -3.970404413101018104 ) ) ;
#14596=CARTESIAN_POINT ( 'NONE',  ( 27.85548922659574700, -68.67521603617417725, 4.260811380381850810 ) ) ;
#14602=CARTESIAN_POINT ( 'NONE',  ( 30.71459926079771918, -62.29356353674184987, -3.270869388464555438 ) ) ;
#14603=ORIENTED_EDGE ( 'NONE', *, *, #13408, .T. ) ;
#14616=DIRECTION ( 'NONE',  ( 0.000000000000000000, 1.000000000000000000, 0.000000000000000000 ) ) ;
#14617=( BOUNDED_SURFACE ( )  B_SPLINE_SURFACE ( 3, 2, ( 
 ( #840, #8851, #8931 ),
 ( #8007, #14701, #14850 ),
 ( #13622, #12470, #4300 ),
 ( #5549, #918, #4153 ),
 ( #10399, #15094, #4543 ),
 ( #9245, #13933, #5711 ),
 ( #10880, #1405, #10801 ),
 ( #10652, #113, #14191 ),
 ( #7332, #3934, #8347 ),
 ( #4798, #3713, #3860 ),
 ( #338, #14487, #1333 ),
 ( #14265, #5030, #3793 ),
 ( #12020, #14417, #8631 ),
 ( #8562, #11944, #12105 ),
 ( #9581, #2414, #1565 ),
 ( #9497, #9735, #6114 ),
 ( #7108, #261, #10954 ),
 ( #2639, #1486, #6191 ),
 ( #13260, #8498, #11795 ),
 ( #2714, #1251, #13183 ),
 ( #5965, #8422, #10721 ),
 ( #6264, #6037, #3646 ),
 ( #13115, #2570, #7408 ),
 ( #13038, #4948, #2486 ) ),
 .UNSPECIFIED., .F., .F., .T. ) 
 B_SPLINE_SURFACE_WITH_KNOTS ( ( 4, 2, 2, 2, 2, 2, 2, 2, 2, 2, 2, 4 ),
 ( 3, 3 ),
 ( 0.000000000000000000, 0.0007560557787111729612, 0.001512111557422345922, 0.001890139446777932240, 0.002268167336133518775, 0.003024223114844691845, 0.003402251004200278379, 0.003780278893555864481, 0.004158306782911451449, 0.004536334672267037550, 0.005292390450978210620, 0.006048446229689383689 ),
 ( 0.000000000000000000, 1.000000000000000000 ),
 .UNSPECIFIED. ) 
 GEOMETRIC_REPRESENTATION_ITEM ( )  RATIONAL_B_SPLINE_SURFACE ( (
 ( 1.000000000000000000, 0.8250833044923658877, 1.000000000000000000),
 ( 1.000000000000000000, 0.8244629924933467580, 1.000000000000000000),
 ( 1.000000000000000000, 0.8228453557281663056, 1.000000000000000000),
 ( 1.000000000000000000, 0.8179470878186148042, 1.000000000000000000),
 ( 1.000000000000000000, 0.8146336382298167145, 1.000000000000000000),
 ( 1.000000000000000000, 0.8088012687532515343, 1.000000000000000000),
 ( 1.000000000000000000, 0.8067039814524846753, 1.000000000000000000),
 ( 1.000000000000000000, 0.8022097056812232951, 1.000000000000000000),
 ( 1.000000000000000000, 0.7997977307760982812, 1.000000000000000000),
 ( 1.000000000000000000, 0.7922670365021369232, 1.000000000000000000),
 ( 1.000000000000000000, 0.7868330064134674284, 1.000000000000000000),
 ( 1.000000000000000000, 0.7779933494262166738, 1.000000000000000000),
 ( 1.000000000000000000, 0.7749217965225499993, 1.000000000000000000),
 ( 1.000000000000000000, 0.7686646892562868372, 1.000000000000000000),
 ( 1.000000000000000000, 0.7654626812325054930, 1.000000000000000000),
 ( 1.000000000000000000, 0.7588889951604184114, 1.000000000000000000),
 ( 1.000000000000000000, 0.7555173610299135145, 1.000000000000000000),
 ( 1.000000000000000000, 0.7485733441930104703, 1.000000000000000000),
 ( 1.000000000000000000, 0.7449916546359187652, 1.000000000000000000),
 ( 1.000000000000000000, 0.7341394734815585021, 1.000000000000000000),
 ( 1.000000000000000000, 0.7266881283996446950, 1.000000000000000000),
 ( 1.000000000000000000, 0.7111189506802038096, 1.000000000000000000),
 ( 1.000000000000000000, 0.7029851397915697353, 1.000000000000000000),
 ( 1.000000000000000000, 0.6947298545087505772, 1.000000000000000000) ) ) 
 REPRESENTATION_ITEM ( '' )  SURFACE ( )  );
#14623=CARTESIAN_POINT ( 'NONE',  ( 14.04356807544018437, -66.53205946168881724, -4.446982897617355768 ) ) ;
#14625=CARTESIAN_POINT ( 'NONE',  ( 14.38963276113425138, -69.39711819508849544, -4.502057496415714510 ) ) ;
#14629=EDGE_CURVE ( 'NONE', #304, #8543, #12755, .T. ) ;
#14630=DIRECTION ( 'NONE',  ( 0.000000000000000000, 1.000000000000000000, -0.000000000000000000 ) ) ;
#14631=DIRECTION ( 'NONE',  ( -0.9744556954135537019, 0.2245798247307348450, 0.000000000000000000 ) ) ;
#14649=ORIENTED_EDGE ( 'NONE', *, *, #12996, .T. ) ;
#14655=CARTESIAN_POINT ( 'NONE',  ( 10.03094031226078897, -52.93050895625587771, 3.457921359511975989 ) ) ;
#14663=CARTESIAN_POINT ( 'NONE',  ( 10.23047706855496664, -60.71197230342421136, 3.050751728647393080 ) ) ;
#14664=ORIENTED_EDGE ( 'NONE', *, *, #1349, .T. ) ;
#14673=AXIS2_PLACEMENT_3D ( 'NONE', #1993, #12628, #3231 ) ;
#14674=EDGE_CURVE ( 'NONE', #14491, #14799, #790, .T. ) ;
#14679=DIRECTION ( 'NONE',  ( -0.000000000000000000, -0.000000000000000000, -1.000000000000000000 ) ) ;
#14680=B_SPLINE_CURVE_WITH_KNOTS ( 'NONE', 3,
 ( #2291, #12995, #3525, #13065, #13906, #15140, #2522, #10601, #4826, #7212 ),
 .UNSPECIFIED., .F., .F.,
 ( 4, 2, 2, 2, 4 ),
 ( 7.866258489732282489E-18, 0.002320432257317498782, 0.004640864514634989758, 0.006961296771952480734, 0.009281729029269972578 ),
 .UNSPECIFIED. ) ;
#14689=VERTEX_POINT ( 'NONE', #1434 ) ;
#14690=ORIENTED_EDGE ( 'NONE', *, *, #13545, .F. ) ;
#14696=EDGE_LOOP ( 'NONE', ( #14468, #13384 ) ) ;
#14701=CARTESIAN_POINT ( 'NONE',  ( 33.59357299507875894, -57.17459804182058036, -2.501046471589234876 ) ) ;
#14709=CARTESIAN_POINT ( 'NONE',  ( 28.81202928791190843, -63.78335865426900142, -4.036657210498111326 ) ) ;
#14710=( BOUNDED_SURFACE ( )  B_SPLINE_SURFACE ( 3, 2, ( 
 ( #4635, #1477, #8261 ),
 ( #7245, #7018, #11864 ),
 ( #12953, #9649, #104 ),
 ( #3783, #4790, #9485 ) ),
 .UNSPECIFIED., .F., .F., .F. ) 
 B_SPLINE_SURFACE_WITH_KNOTS ( ( 4, 4 ),
 ( 3, 3 ),
 ( 0.000000000000000000, 0.001771943201165739230 ),
 ( 0.000000000000000000, 1.000000000000000000 ),
 .UNSPECIFIED. ) 
 GEOMETRIC_REPRESENTATION_ITEM ( )  RATIONAL_B_SPLINE_SURFACE ( (
 ( 1.000000000000000000, 0.8250833044923668869, 1.000000000000000000),
 ( 1.000000000000000000, 0.8269348987755763547, 1.000000000000000000),
 ( 1.000000000000000000, 0.8288551047899433977, 1.000000000000000000),
 ( 1.000000000000000000, 0.8308543624379425285, 1.000000000000000000) ) ) 
 REPRESENTATION_ITEM ( '' )  SURFACE ( )  );
#14714=CARTESIAN_POINT ( 'NONE',  ( 33.12442989620986822, -59.21224831720011395, -1.832439066039627251 ) ) ;
#14717=DIRECTION ( 'NONE',  ( 0.000000000000000000, 0.000000000000000000, -1.000000000000000000 ) ) ;
#14725=FACE_OUTER_BOUND ( 'NONE', #14211, .T. ) ;
#14731=CARTESIAN_POINT ( 'NONE',  ( 9.841896756782944067, -61.30062302791114348, 2.840369378987775306 ) ) ;
#14734=CARTESIAN_POINT ( 'NONE',  ( 33.52235686305655804, -57.48563641131178770, -1.816685854991392457 ) ) ;
#14742=CARTESIAN_POINT ( 'NONE',  ( 32.06570158546600169, -54.31552982368702231, -3.256647958671372134 ) ) ;
#14743=EDGE_LOOP ( 'NONE', ( #12649, #10922, #11006, #10577, #9040, #11512, #13731, #13093 ) ) ;
#14750=CARTESIAN_POINT ( 'NONE',  ( 27.85761975137823043, -68.67486713608998627, -3.656664647162143122 ) ) ;
#14752=CARTESIAN_POINT ( 'NONE',  ( 11.55751249766752764, -53.31348408104178560, -3.971884189131345444 ) ) ;
#14757=CARTESIAN_POINT ( 'NONE',  ( 10.00023835250150483, -61.42570632716525125, -2.132522520905374197 ) ) ;
#14759=ORIENTED_EDGE ( 'NONE', *, *, #12773, .T. ) ;
#14776=DIRECTION ( 'NONE',  ( 0.000000000000000000, -1.000000000000000000, 0.000000000000000000 ) ) ;
#14777=CARTESIAN_POINT ( 'NONE',  ( 10.87912556055781543, -61.22098757970782401, -3.286659897583100065 ) ) ;
#14793=CARTESIAN_POINT ( 'NONE',  ( 32.98177247948689939, -56.83166877439235520, 2.758334070755382950 ) ) ;
#14799=VERTEX_POINT ( 'NONE', #1727 ) ;
#14801=PLANE ( 'NONE',  #13815 ) ;
#14809=CARTESIAN_POINT ( 'NONE',  ( 12.96675353036119738, -65.20845675887582615, 3.989712384462641204 ) ) ;
#14810=B_SPLINE_CURVE_WITH_KNOTS ( 'NONE', 3,
 ( #9350, #10806, #10581, #1412, #2644, #1102, #13043, #7263, #7186, #9665 ),
 .UNSPECIFIED., .F., .F.,
 ( 4, 2, 2, 2, 4 ),
 ( 4.399029233930689259E-17, 0.0004995983118108281032, 0.0009991966236216121879, 0.001498794935432396164, 0.001998393247243180140 ),
 .UNSPECIFIED. ) ;
#14811=CARTESIAN_POINT ( 'NONE',  ( 9.624670876293347277, -53.24145049768178950, 2.425475548247288948 ) ) ;
#14812=DIRECTION ( 'NONE',  ( 0.000000000000000000, 1.000000000000000000, -0.000000000000000000 ) ) ;
#14818=ORIENTED_EDGE ( 'NONE', *, *, #5591, .T. ) ;
#14827=CIRCLE ( 'NONE', #12371, 7.000000000000000000 ) ;
#14833=ORIENTED_EDGE ( 'NONE', *, *, #5655, .F. ) ;
#14835=CARTESIAN_POINT ( 'NONE',  ( 8.788876864333699857, -56.07566194134416548, -2.832314198476005629 ) ) ;
#14847=CARTESIAN_POINT ( 'NONE',  ( 11.54983932419131243, -53.31455134687481490, -3.969134470563519645 ) ) ;
#14848=ORIENTED_EDGE ( 'NONE', *, *, #14629, .F. ) ;
#14850=CARTESIAN_POINT ( 'NONE',  ( 33.59732214446785292, -57.16036077483331468, -1.814506011343099523 ) ) ;
#14851=CARTESIAN_POINT ( 'NONE',  ( 13.39143123690972281, -66.31583591551519419, -4.137138225905224509 ) ) ;
#14859=CARTESIAN_POINT ( 'NONE',  ( 28.61048634131497792, -64.14571591460358491, -4.111538053172250073 ) ) ;
#14869=CARTESIAN_POINT ( 'NONE',  ( 32.82077387253592349, -55.58469383501343941, 2.908670588548392999 ) ) ;
#14872=ORIENTED_EDGE ( 'NONE', *, *, #1694, .F. ) ;
#14883=B_SPLINE_CURVE_WITH_KNOTS ( 'NONE', 3,
 ( #10856, #3695, #91, #316 ),
 .UNSPECIFIED., .F., .F.,
 ( 4, 4 ),
 ( 0.000000000000000000, 0.001771361151111836311 ),
 .UNSPECIFIED. ) ;
#14890=ORIENTED_EDGE ( 'NONE', *, *, #6126, .F. ) ;
#14891=CARTESIAN_POINT ( 'NONE',  ( 18.61871093201827421, -52.24929059928630437, -5.564967562786278243 ) ) ;
#14896=CARTESIAN_POINT ( 'NONE',  ( 14.38963276113425138, -69.39711819508849544, -4.502057496415714510 ) ) ;
#14898=DIRECTION ( 'NONE',  ( 0.000000000000000000, 1.000000000000000000, -0.000000000000000000 ) ) ;
#14905=CARTESIAN_POINT ( 'NONE',  ( 8.756240387056642760, -56.32851134755706113, -2.801743212233170688 ) ) ;
#14916=ORIENTED_EDGE ( 'NONE', *, *, #55, .F. ) ;
#14923=VERTEX_POINT ( 'NONE', #12500 ) ;
#14932=CIRCLE ( 'NONE', #1666, 31.00000000000000000 ) ;
#14934=CARTESIAN_POINT ( 'NONE',  ( 35.08843044364380859, -47.02811197266221654, 2.732446379177822848 ) ) ;
#14938=CARTESIAN_POINT ( 'NONE',  ( 33.59375882623609044, -57.17378631614185736, 2.501045389179021861 ) ) ;
#14941=CARTESIAN_POINT ( 'NONE',  ( 19.97461805067967333, -82.24929059928629727, 4.000000000000001776 ) ) ;
#14948=ORIENTED_EDGE ( 'NONE', *, *, #13357, .T. ) ;
#14954=CARTESIAN_POINT ( 'NONE',  ( 19.97461805067967688, -85.24929059928631148, -4.000000000000000888 ) ) ;
#14957=ORIENTED_EDGE ( 'NONE', *, *, #13545, .T. ) ;
#14962=CARTESIAN_POINT ( 'NONE',  ( 8.091875466796901506, -56.24057709915800274, 1.858739038532483123 ) ) ;
#14967=DIRECTION ( 'NONE',  ( -0.000000000000000000, 1.000000000000000000, -0.000000000000000000 ) ) ;
#14968=CARTESIAN_POINT ( 'NONE',  ( 10.00023835250150661, -61.42570632716525836, 2.132522520905367980 ) ) ;
#14970=DIRECTION ( 'NONE',  ( 0.000000000000000000, 0.000000000000000000, 1.000000000000000000 ) ) ;
#14971=CARTESIAN_POINT ( 'NONE',  ( 32.52281604437752804, -59.06479067038043240, 2.757123406423070744 ) ) ;
#14972=DIRECTION ( 'NONE',  ( 0.9744556954135545901, 0.2245798247307308204, 0.000000000000000000 ) ) ;
#14973=CARTESIAN_POINT ( 'NONE',  ( 9.488545476451129446, -59.84602720838573475, 2.809343037843349045 ) ) ;
#14982=CARTESIAN_POINT ( 'NONE',  ( 12.22773363228717614, -62.74876579108499897, -3.782929430830273443 ) ) ;
#14986=CARTESIAN_POINT ( 'NONE',  ( 21.74884261173415467, -96.56299909827106376, 4.000000000000001776 ) ) ;
#14990=CIRCLE ( 'NONE', #8369, 7.000000000000000000 ) ;
#14992=CARTESIAN_POINT ( 'NONE',  ( 8.199792978590132009, -57.47994873761392398, -2.501453769636599045 ) ) ;
#15004=ORIENTED_EDGE ( 'NONE', *, *, #7032, .F. ) ;
#15022=DIRECTION ( 'NONE',  ( -0.000000000000000000, 1.000000000000000000, -0.000000000000000000 ) ) ;
#15032=CARTESIAN_POINT ( 'NONE',  ( 31.30110669430510129, -53.71233130651034315, 3.555899869131480706 ) ) ;
#15037=ORIENTED_EDGE ( 'NONE', *, *, #13357, .F. ) ;
#15038=CARTESIAN_POINT ( 'NONE',  ( 31.96811279043434340, -60.26979819505955760, 2.885043711492953467 ) ) ;
#15045=CARTESIAN_POINT ( 'NONE',  ( 24.62796245282055452, -82.24929059928629727, -1.347403282660978752 ) ) ;
#15051=CARTESIAN_POINT ( 'NONE',  ( 31.62073844763337149, -60.61171897230391892, 3.004288329735560925 ) ) ;
#15055=CIRCLE ( 'NONE', #508, 1.000000000000000000 ) ;
#15056=PLANE ( 'NONE',  #11480 ) ;
#15058=ORIENTED_EDGE ( 'NONE', *, *, #10927, .F. ) ;
#15059=CARTESIAN_POINT ( 'NONE',  ( 8.859806296821686189, -57.78392871910184425, -2.727962224264455227 ) ) ;
#15065=CARTESIAN_POINT ( 'NONE',  ( 13.47628073630851731, -64.89641169172402613, -4.245552436241592176 ) ) ;
#15066=CARTESIAN_POINT ( 'NONE',  ( 17.87818865416384995, -64.01730164816855506, -6.333338579777395339 ) ) ;
#15069=CARTESIAN_POINT ( 'NONE',  ( 18.61871093201827065, -52.24929059928630437, -5.564967562786285349 ) ) ;
#15072=CIRCLE ( 'NONE', #11872, 3.999999999999999112 ) ;
#15076=CARTESIAN_POINT ( 'NONE',  ( 8.142427707716008101, -55.84923954203681973, -1.895000442031717913 ) ) ;
#15080=DIRECTION ( 'NONE',  ( 0.000000000000000000, 0.000000000000000000, -1.000000000000000000 ) ) ;
#15091=VERTEX_POINT ( 'NONE', #9505 ) ;
#15092=CARTESIAN_POINT ( 'NONE',  ( 20.86173033120691045, -53.24929059928630437, 0.000000000000000000 ) ) ;
#15094=CARTESIAN_POINT ( 'NONE',  ( 33.60245346892040885, -55.93345933723782792, -2.599599694949141337 ) ) ;
#15095=CARTESIAN_POINT ( 'NONE',  ( 23.47858629692699495, -52.24929059928630437, 6.492462156583981958 ) ) ;
#15096=CARTESIAN_POINT ( 'NONE',  ( 31.77253520366416950, -63.13950256936100658, 2.713503986087918651 ) ) ;
#15097=ORIENTED_EDGE ( 'NONE', *, *, #1365, .F. ) ;
#15112=CARTESIAN_POINT ( 'NONE',  ( 18.61871093201827421, -52.24929059928630437, -5.564967562786278243 ) ) ;
#15117=CARTESIAN_POINT ( 'NONE',  ( 24.36188411769309781, -73.69234276600508338, -6.062089035220971311 ) ) ;
#15133=CARTESIAN_POINT ( 'NONE',  ( 12.93509704890846557, -54.57042255619801097, -4.214900875586402584 ) ) ;
#15135=CARTESIAN_POINT ( 'NONE',  ( 8.201103799357262858, -57.48563641131178770, 1.816685854991387794 ) ) ;
#15137=CARTESIAN_POINT ( 'NONE',  ( 27.80179776399110736, -69.39711819508849544, 3.972674503026243809 ) ) ;
#15140=CARTESIAN_POINT ( 'NONE',  ( 13.15381962123460191, -65.59433601606468756, -3.409308316089461055 ) ) ;
#15144=CARTESIAN_POINT ( 'NONE',  ( 8.128335720592605895, -55.93948076112146595, -2.601440957440732227 ) ) ;
#15148=AXIS2_PLACEMENT_3D ( 'NONE', #3702, #2400, #11861 ) ;
#15162=ORIENTED_EDGE ( 'NONE', *, *, #1810, .T. ) ;
#15183=DIRECTION ( 'NONE',  ( -0.000000000000000000, 1.000000000000000000, -0.000000000000000000 ) ) ;
#15184=TOROIDAL_SURFACE ( 'NONE', #1652, 6.000000000000000000, 1.000000000000000000 ) ;
#15187=CARTESIAN_POINT ( 'NONE',  ( 10.00023835250150483, -61.42570632716525125, 2.500000000000000000 ) ) ;
#15191=VERTEX_POINT ( 'NONE', #5259 ) ;
#15195=CARTESIAN_POINT ( 'NONE',  ( 13.86173033120691223, -69.39711819508849544, 2.500000000000000000 ) ) ;
#15200=EDGE_CURVE ( 'NONE', #14923, #3720, #10241, .T. ) ;
#15206=CARTESIAN_POINT ( 'NONE',  ( 31.78593137074030395, -54.06014836395551271, 3.368555242453529885 ) ) ;
#15208=CARTESIAN_POINT ( 'NONE',  ( 18.00340353970562646, -60.79495753919547241, -6.390225278801568543 ) ) ;
#15214=ORIENTED_EDGE ( 'NONE', *, *, #1475, .F. ) ;
#15215=CARTESIAN_POINT ( 'NONE',  ( 12.36791015745245836, -56.52532528994181860, 2.500000000000000000 ) ) ;
#15224=CARTESIAN_POINT ( 'NONE',  ( 53.81626139532630049, -82.24929059928629727, -11.78977872328356646 ) ) ;
#15266=COLOUR_RGB('Black',0.12,0.14,0.17);
#15267=FILL_AREA_STYLE_COLOUR('',#15266);
#15268=FILL_AREA_STYLE('',(#15267));
#15269=SURFACE_STYLE_FILL_AREA(#15268);
#15270=SURFACE_SIDE_STYLE('',(#15269));
#15271=SURFACE_STYLE_USAGE(.BOTH.,#15270);
#15272=PRESENTATION_STYLE_ASSIGNMENT((#15271));
ENDSEC;
END-ISO-10303-21;
